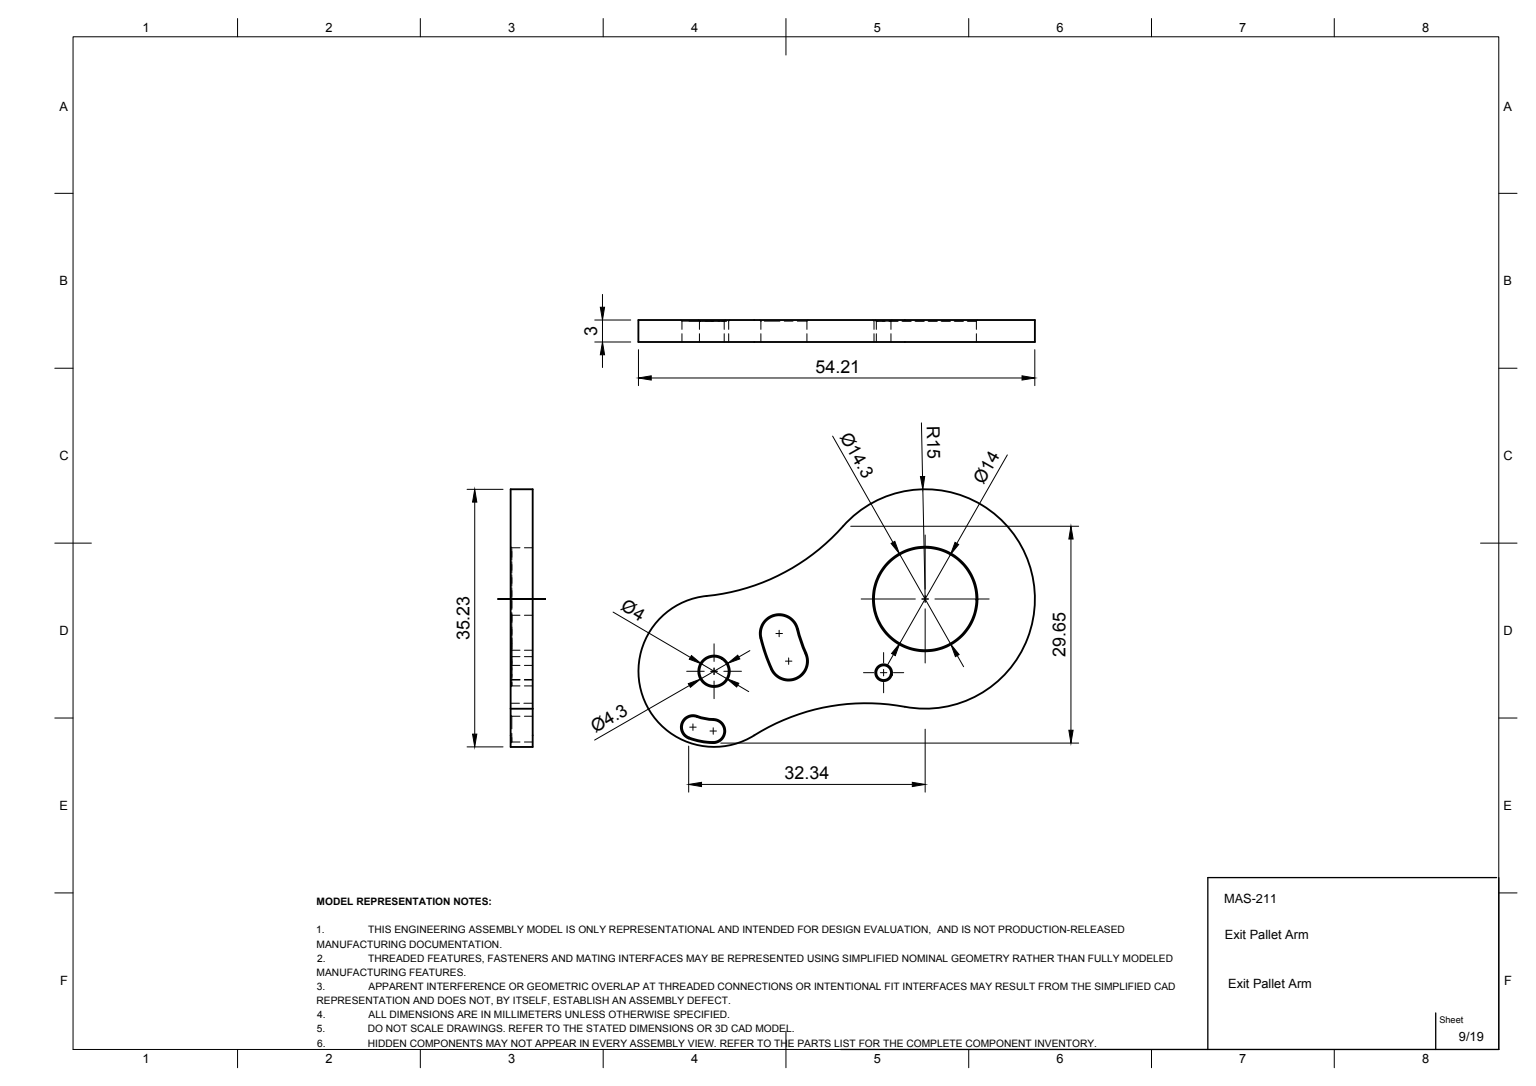
ISO-10303-21;
HEADER;
FILE_DESCRIPTION(
 (''),
 '2;1');
FILE_NAME ( 'Exit Pallet Arm.step', '2026-10-05T20:07:59+06:00', ( '' ), ( '' ), 'STEP AP214', 'Unspecified', '' );
FILE_SCHEMA (('AUTOMOTIVE_DESIGN { 1 0 10303 214 3 1 1 }'));
ENDSEC;
DATA;
#10=MECHANICAL_DESIGN_GEOMETRIC_PRESENTATION_REPRESENTATION('',(#326),#196741);
#135=ELLIPSE('',#8916,15.4840898354346,13.4083590350904) ;
#136=ELLIPSE('',#8917,20.0777465510709,17.3862071407216) ;
#137=ELLIPSE('',#8918,8.52758470717412,7.38293667736543) ;
#138=ELLIPSE('',#8919,5.66235729881268,4.90229438477269) ;
#326=STYLED_ITEM('',(#196765),#345) ;
#345=MANIFOLD_SOLID_BREP('Exit Pallet Arm',#8722) ;
#387=PLANE('',#8903) ;
#388=PLANE('',#8915) ;
#576=FACE_BOUND('',#1481,.T.) ;
#577=FACE_BOUND('',#1482,.T.) ;
#578=FACE_BOUND('',#1483,.T.) ;
#579=FACE_BOUND('',#1484,.T.) ;
#580=FACE_BOUND('',#1485,.T.) ;
#581=FACE_BOUND('',#1487,.T.) ;
#582=FACE_BOUND('',#1488,.T.) ;
#583=FACE_BOUND('',#1489,.T.) ;
#584=FACE_BOUND('',#1490,.T.) ;
#585=FACE_BOUND('',#1491,.T.) ;
#664=CIRCLE('',#8892,28.7407375552556) ;
#665=CIRCLE('',#8893,28.7407375552556) ;
#666=CIRCLE('',#8895,15.) ;
#667=CIRCLE('',#8896,15.) ;
#668=CIRCLE('',#8898,28.7407375552573) ;
#669=CIRCLE('',#8899,28.7407375552573) ;
#670=CIRCLE('',#8901,10.3432265401781) ;
#671=CIRCLE('',#8902,10.3432265401781) ;
#672=CIRCLE('',#8904,2.) ;
#673=CIRCLE('',#8905,23.0149881946393) ;
#674=CIRCLE('',#8906,2.4999999999999) ;
#675=CIRCLE('',#8907,18.0149881946822) ;
#676=CIRCLE('',#8908,2.49999999999984) ;
#677=CIRCLE('',#8909,7.) ;
#678=CIRCLE('',#8910,1.49999999999999) ;
#679=CIRCLE('',#8911,6.67161327010524) ;
#680=CIRCLE('',#8912,1.49999999999977) ;
#681=CIRCLE('',#8913,9.67161327008901) ;
#682=CIRCLE('',#8914,0.999999999999985) ;
#683=CIRCLE('',#8921,2.00000000000002) ;
#684=CIRCLE('',#8924,18.0149881946818) ;
#685=CIRCLE('',#8928,7.) ;
#686=CIRCLE('',#8932,6.67161327010476) ;
#846=B_SPLINE_SURFACE_WITH_KNOTS('',3,1,((#113566,#113567),(#113568,#113569),
(#113570,#113571),(#113572,#113573),(#113574,#113575),(#113576,#113577),
(#113578,#113579),(#113580,#113581),(#113582,#113583),(#113584,#113585),
(#113586,#113587),(#113588,#113589),(#113590,#113591),(#113592,#113593),
(#113594,#113595),(#113596,#113597),(#113598,#113599),(#113600,#113601),
(#113602,#113603)),.UNSPECIFIED.,.T.,.F.,.F.,(4,1,1,1,1,1,1,1,1,1,1,1,1,
1,1,1,4),(2,2),(0.,0.844281694673181,1.68856338934636,2.5328450840081,3.37712677866985,
4.22140847333585,5.06569016800186,5.90997186266359,6.75425355732532,7.59853525198361,
8.44281694664191,9.28709864130793,10.131380335974,10.9756620306357,11.8199437252974,
12.6642254199629,13.5085071146283),(-0.0112712723182462,0.214916064351496),
 .UNSPECIFIED.) ;
#847=B_SPLINE_SURFACE_WITH_KNOTS('',3,1,((#113605,#113606),(#113607,#113608),
(#113609,#113610),(#113611,#113612),(#113613,#113614),(#113615,#113616),
(#113617,#113618),(#113619,#113620),(#113621,#113622),(#113623,#113624),
(#113625,#113626)),.UNSPECIFIED.,.F.,.F.,.F.,(4,1,1,1,1,1,1,1,4),(2,2),
(0.,1.04064620349252,2.08129240698504,3.12193860704037,4.16258480709569,
5.20323100714621,6.24387720719672,7.28452341068925,8.32516961418178),(0.,
0.214915892305322),.UNSPECIFIED.) ;
#848=B_SPLINE_SURFACE_WITH_KNOTS('',3,1,((#113629,#113630),(#113631,#113632),
(#113633,#113634),(#113635,#113636)),.UNSPECIFIED.,.F.,.F.,.F.,(4,4),(2,
2),(-1.11022302462516E-16,3.4846841528001),(0.,0.212356567860235),
 .UNSPECIFIED.) ;
#849=B_SPLINE_SURFACE_WITH_KNOTS('',3,1,((#113638,#113639),(#113640,#113641),
(#113642,#113643),(#113644,#113645),(#113646,#113647),(#113648,#113649),
(#113650,#113651),(#113652,#113653),(#113654,#113655),(#113656,#113657),
(#113658,#113659)),.UNSPECIFIED.,.F.,.F.,.F.,(4,1,1,1,1,1,1,1,4),(2,2),
(0.,1.04062614942688,2.08125229885376,3.12187844827613,4.1625045976985,
5.20313074711665,6.24375689653479,7.28438304596787,8.32500919540094),(0.,
0.214916063344399),.UNSPECIFIED.) ;
#850=B_SPLINE_SURFACE_WITH_KNOTS('',3,1,((#113661,#113662),(#113663,#113664),
(#113665,#113666),(#113667,#113668)),.UNSPECIFIED.,.F.,.F.,.F.,(4,4),(2,
2),(-1.11022302462516E-16,4.5184839002944),(-6.99189761287855E-5,0.212356567829033),
 .UNSPECIFIED.) ;
#851=B_SPLINE_SURFACE_WITH_KNOTS('',3,1,((#113669,#113670),(#113671,#113672),
(#113673,#113674),(#113675,#113676),(#113677,#113678),(#113679,#113680),
(#113681,#113682),(#113683,#113684),(#113685,#113686),(#113687,#113688),
(#113689,#113690),(#113691,#113692),(#113693,#113694),(#113695,#113696),
(#113697,#113698),(#113699,#113700),(#113701,#113702),(#113703,#113704),
(#113705,#113706)),.UNSPECIFIED.,.T.,.F.,.F.,(4,1,1,1,1,1,1,1,1,1,1,1,1,
1,1,1,4),(2,2),(0.,2.69519445779222,5.61545499238395,8.53571552697321,11.2309099847624,
13.9261044425516,16.8463649771433,19.7666255117326,22.4618199695217,25.1570144273109,
28.0772749619002,30.9975354964919,33.692729954281,36.3879244120702,39.3081849466595,
42.2284454812513,44.9236399390404),(-0.0215150649611441,0.215150649611441),
 .UNSPECIFIED.) ;
#852=B_SPLINE_SURFACE_WITH_KNOTS('',3,1,((#113708,#113709),(#113710,#113711),
(#113712,#113713),(#113714,#113715)),.UNSPECIFIED.,.F.,.F.,.F.,(4,4),(2,
2),(-1.20032081259135E-14,3.40704145701401),(-0.000292137134752522,0.212844506430324),
 .UNSPECIFIED.) ;
#853=B_SPLINE_SURFACE_WITH_KNOTS('',3,1,((#113718,#113719),(#113720,#113721),
(#113722,#113723),(#113724,#113725),(#113726,#113727),(#113728,#113729),
(#113730,#113731),(#113732,#113733),(#113734,#113735)),.UNSPECIFIED.,.F.,
 .F.,.F.,(4,1,1,1,1,1,4),(2,2),(0.,1.2958739093245,1.94381087119137,2.59174783305825,
3.23968479492247,3.88762175678669,5.18349566611894),(0.,0.218727515290808),
 .UNSPECIFIED.) ;
#854=B_SPLINE_SURFACE_WITH_KNOTS('',3,1,((#113737,#113738),(#113739,#113740),
(#113741,#113742),(#113743,#113744)),.UNSPECIFIED.,.F.,.F.,.F.,(4,4),(2,
2),(0.,2.26229870547723),(0.,0.212844507129729),.UNSPECIFIED.) ;
#855=B_SPLINE_SURFACE_WITH_KNOTS('',3,1,((#113746,#113747),(#113748,#113749),
(#113750,#113751),(#113752,#113753),(#113754,#113755),(#113756,#113757),
(#113758,#113759),(#113760,#113761),(#113762,#113763)),.UNSPECIFIED.,.F.,
 .F.,.F.,(4,1,1,1,1,1,4),(2,2),(0.,1.29587422179652,1.94381133989956,2.5917484580026,
3.23968557610299,3.88762269420339,5.18349691602093),(0.,0.21872751905286),
 .UNSPECIFIED.) ;
#856=B_SPLINE_SURFACE_WITH_KNOTS('',3,1,((#113764,#113765),(#113766,#113767),
(#113768,#113769),(#113770,#113771),(#113772,#113773),(#113774,#113775),
(#113776,#113777),(#113778,#113779),(#113780,#113781),(#113782,#113783),
(#113784,#113785)),.UNSPECIFIED.,.T.,.F.,.F.,(4,1,1,1,1,1,1,1,4),(2,2),
(0.,0.903185063809554,1.80637013757091,2.70955520128371,3.61274027504511,
4.51592534880276,5.4191104125156,6.32229548627704,7.22548054998985),(0.,
0.223990409920864),.UNSPECIFIED.) ;
#981=FACE_OUTER_BOUND('',#1476,.T.) ;
#982=FACE_OUTER_BOUND('',#1477,.T.) ;
#983=FACE_OUTER_BOUND('',#1478,.T.) ;
#984=FACE_OUTER_BOUND('',#1479,.T.) ;
#985=FACE_OUTER_BOUND('',#1480,.T.) ;
#986=FACE_OUTER_BOUND('',#1486,.T.) ;
#987=FACE_OUTER_BOUND('',#1492,.T.) ;
#988=FACE_OUTER_BOUND('',#1493,.T.) ;
#989=FACE_OUTER_BOUND('',#1494,.T.) ;
#990=FACE_OUTER_BOUND('',#1495,.T.) ;
#991=FACE_OUTER_BOUND('',#1496,.T.) ;
#992=FACE_OUTER_BOUND('',#1497,.T.) ;
#993=FACE_OUTER_BOUND('',#1498,.T.) ;
#994=FACE_OUTER_BOUND('',#1499,.T.) ;
#995=FACE_OUTER_BOUND('',#1500,.T.) ;
#996=FACE_OUTER_BOUND('',#1501,.T.) ;
#997=FACE_OUTER_BOUND('',#1502,.T.) ;
#998=FACE_OUTER_BOUND('',#1503,.T.) ;
#999=FACE_OUTER_BOUND('',#1504,.T.) ;
#1000=FACE_OUTER_BOUND('',#1505,.T.) ;
#1001=FACE_OUTER_BOUND('',#1506,.T.) ;
#1002=FACE_OUTER_BOUND('',#1507,.T.) ;
#1003=FACE_OUTER_BOUND('',#1508,.T.) ;
#1004=FACE_OUTER_BOUND('',#1509,.T.) ;
#1005=FACE_OUTER_BOUND('',#1510,.T.) ;
#1006=FACE_OUTER_BOUND('',#1511,.T.) ;
#1007=FACE_OUTER_BOUND('',#1512,.T.) ;
#1008=FACE_OUTER_BOUND('',#1513,.T.) ;
#1476=EDGE_LOOP('',(#6216,#6217,#6218,#6219)) ;
#1477=EDGE_LOOP('',(#6220,#6221,#6222,#6223)) ;
#1478=EDGE_LOOP('',(#6224,#6225,#6226,#6227)) ;
#1479=EDGE_LOOP('',(#6228,#6229,#6230,#6231)) ;
#1480=EDGE_LOOP('',(#6232,#6233,#6234,#6235)) ;
#1481=EDGE_LOOP('',(#6236)) ;
#1482=EDGE_LOOP('',(#6237,#6238,#6239,#6240)) ;
#1483=EDGE_LOOP('',(#6241)) ;
#1484=EDGE_LOOP('',(#6242,#6243,#6244,#6245)) ;
#1485=EDGE_LOOP('',(#6246)) ;
#1486=EDGE_LOOP('',(#6247,#6248,#6249,#6250)) ;
#1487=EDGE_LOOP('',(#6251)) ;
#1488=EDGE_LOOP('',(#6252,#6253,#6254,#6255)) ;
#1489=EDGE_LOOP('',(#6256)) ;
#1490=EDGE_LOOP('',(#6257,#6258,#6259,#6260)) ;
#1491=EDGE_LOOP('',(#6261)) ;
#1492=EDGE_LOOP('',(#6262,#6263,#6264,#6265)) ;
#1493=EDGE_LOOP('',(#6266,#6267,#6268,#6269)) ;
#1494=EDGE_LOOP('',(#6270,#6271,#6272,#6273)) ;
#1495=EDGE_LOOP('',(#6274,#6275,#6276,#6277)) ;
#1496=EDGE_LOOP('',(#6278,#6279,#6280,#6281)) ;
#1497=EDGE_LOOP('',(#6282,#6283,#6284,#6285)) ;
#1498=EDGE_LOOP('',(#6286,#6287,#6288,#6289)) ;
#1499=EDGE_LOOP('',(#6290,#6291,#6292,#6293)) ;
#1500=EDGE_LOOP('',(#6294,#6295,#6296,#6297)) ;
#1501=EDGE_LOOP('',(#6298,#6299,#6300,#6301)) ;
#1502=EDGE_LOOP('',(#6302,#6303,#6304,#6305)) ;
#1503=EDGE_LOOP('',(#6306,#6307,#6308,#6309)) ;
#1504=EDGE_LOOP('',(#6310,#6311,#6312,#6313)) ;
#1505=EDGE_LOOP('',(#6314,#6315,#6316,#6317)) ;
#1506=EDGE_LOOP('',(#6318,#6319,#6320,#6321)) ;
#1507=EDGE_LOOP('',(#6322,#6323,#6324,#6325)) ;
#1508=EDGE_LOOP('',(#6326,#6327,#6328,#6329)) ;
#1509=EDGE_LOOP('',(#6330,#6331,#6332,#6333)) ;
#1510=EDGE_LOOP('',(#6334,#6335,#6336,#6337)) ;
#1511=EDGE_LOOP('',(#6338,#6339,#6340,#6341)) ;
#1512=EDGE_LOOP('',(#6342,#6343,#6344,#6345)) ;
#1513=EDGE_LOOP('',(#6346,#6347,#6348,#6349)) ;
#1981=LINE('',#113319,#2684) ;
#1982=LINE('',#113322,#2685) ;
#1983=LINE('',#113327,#2686) ;
#1984=LINE('',#113333,#2687) ;
#1985=LINE('',#113469,#2688) ;
#1986=LINE('',#113472,#2689) ;
#1987=LINE('',#113474,#2690) ;
#1988=LINE('',#113488,#2691) ;
#1989=LINE('',#113492,#2692) ;
#1990=LINE('',#113514,#2693) ;
#1991=LINE('',#113517,#2694) ;
#1992=LINE('',#113519,#2695) ;
#1993=LINE('',#113528,#2696) ;
#1994=LINE('',#113540,#2697) ;
#1995=LINE('',#113565,#2698) ;
#1996=LINE('',#113604,#2699) ;
#1997=LINE('',#113627,#2700) ;
#1998=LINE('',#113628,#2701) ;
#1999=LINE('',#113637,#2702) ;
#2000=LINE('',#113660,#2703) ;
#2001=LINE('',#113707,#2704) ;
#2002=LINE('',#113716,#2705) ;
#2003=LINE('',#113717,#2706) ;
#2004=LINE('',#113736,#2707) ;
#2005=LINE('',#113745,#2708) ;
#2006=LINE('',#113786,#2709) ;
#2684=VECTOR('',#9867,10.) ;
#2685=VECTOR('',#9870,10.) ;
#2686=VECTOR('',#9875,10.) ;
#2687=VECTOR('',#9882,10.) ;
#2688=VECTOR('',#9929,2.) ;
#2689=VECTOR('',#9932,10.) ;
#2690=VECTOR('',#9933,10.) ;
#2691=VECTOR('',#9936,10.) ;
#2692=VECTOR('',#9941,10.) ;
#2693=VECTOR('',#9948,6.99999999999998) ;
#2694=VECTOR('',#9951,10.) ;
#2695=VECTOR('',#9952,10.) ;
#2696=VECTOR('',#9955,10.) ;
#2697=VECTOR('',#9958,10.) ;
#2698=VECTOR('',#9965,0.999999999999981) ;
#2699=VECTOR('',#9966,10.) ;
#2700=VECTOR('',#9967,10.) ;
#2701=VECTOR('',#9968,10.) ;
#2702=VECTOR('',#9969,10.) ;
#2703=VECTOR('',#9970,10.) ;
#2704=VECTOR('',#9971,10.) ;
#2705=VECTOR('',#9972,10.) ;
#2706=VECTOR('',#9973,10.) ;
#2707=VECTOR('',#9974,10.) ;
#2708=VECTOR('',#9975,10.) ;
#2709=VECTOR('',#9976,10.) ;
#3419=B_SPLINE_CURVE_WITH_KNOTS('',3,(#113363,#113364,#113365,#113366,#113367,
#113368,#113369,#113370,#113371,#113372,#113373,#113374,#113375,#113376,
#113377,#113378,#113379,#113380,#113381),.UNSPECIFIED.,.T.,.F.,(4,1,1,1,
1,1,1,1,1,1,1,1,1,1,1,1,4),(0.,2.69519445779222,5.61545499238395,8.53571552697321,
11.2309099847624,13.9261044425516,16.8463649771433,19.7666255117326,22.4618199695217,
25.1570144273109,28.0772749619002,30.9975354964919,33.692729954281,36.3879244120702,
39.3081849466595,42.2284454812513,44.9236399390404),.UNSPECIFIED.) ;
#3420=B_SPLINE_CURVE_WITH_KNOTS('',3,(#113384,#113385,#113386,#113387,#113388,
#113389,#113390,#113391,#113392,#113393,#113394),.UNSPECIFIED.,.F.,.F.,
(4,1,1,1,1,1,1,1,4),(0.,1.04064620349252,2.08129240698504,3.12193860704037,
4.16258480709569,5.20323100714621,6.24387720719672,7.28452341068925,8.32516961418178),
 .UNSPECIFIED.) ;
#3421=B_SPLINE_CURVE_WITH_KNOTS('',3,(#113398,#113399,#113400,#113401,#113402,
#113403,#113404,#113405,#113406,#113407,#113408),.UNSPECIFIED.,.F.,.F.,
(4,1,1,1,1,1,1,1,4),(0.,1.04062614942688,2.08125229885376,3.12187844827613,
4.1625045976985,5.20313074711665,6.24375689653479,7.28438304596787,8.32500919540094),
 .UNSPECIFIED.) ;
#3422=B_SPLINE_CURVE_WITH_KNOTS('',3,(#113411,#113412,#113413,#113414,#113415,
#113416,#113417,#113418,#113419,#113420,#113421),.UNSPECIFIED.,.T.,.F.,
(4,1,1,1,1,1,1,1,4),(0.,0.903185063809554,1.80637013757091,2.70955520128371,
3.61274027504511,4.51592534880276,5.4191104125156,6.32229548627704,7.22548054998985),
 .UNSPECIFIED.) ;
#3423=B_SPLINE_CURVE_WITH_KNOTS('',3,(#113426,#113427,#113428,#113429,#113430,
#113431,#113432,#113433,#113434),.UNSPECIFIED.,.F.,.F.,(4,1,1,1,1,1,4),
(0.,1.2958739093245,1.94381087119137,2.59174783305825,3.23968479492247,
3.88762175678669,5.18349566611894),.UNSPECIFIED.) ;
#3424=B_SPLINE_CURVE_WITH_KNOTS('',3,(#113437,#113438,#113439,#113440,#113441,
#113442,#113443,#113444,#113445),.UNSPECIFIED.,.F.,.F.,(4,1,1,1,1,1,4),
(0.,1.29587422179652,1.94381133989956,2.5917484580026,3.23968557610299,
3.88762269420339,5.18349691602093),.UNSPECIFIED.) ;
#3425=B_SPLINE_CURVE_WITH_KNOTS('',3,(#113447,#113448,#113449,#113450,#113451,
#113452,#113453,#113454,#113455,#113456,#113457,#113458,#113459,#113460,
#113461,#113462,#113463,#113464,#113465),.UNSPECIFIED.,.T.,.F.,(4,1,1,1,
1,1,1,1,1,1,1,1,1,1,1,1,4),(0.,0.844281694673181,1.68856338934636,2.5328450840081,
3.37712677866985,4.22140847333585,5.06569016800186,5.90997186266359,6.75425355732532,
7.59853525198361,8.44281694664191,9.28709864130793,10.131380335974,10.9756620306357,
11.8199437252974,12.6642254199629,13.5085071146283),.UNSPECIFIED.) ;
#3426=B_SPLINE_CURVE_WITH_KNOTS('',3,(#113475,#113476,#113477,#113478,#113479,
#113480,#113481,#113482,#113483,#113484,#113485),.UNSPECIFIED.,.F.,.F.,
(4,1,1,1,1,1,1,1,4),(0.,1.04064620349252,2.08129240698504,3.12193860704037,
4.16258480709569,5.20323100714621,6.24387720719672,7.28452341068925,8.32516961418178),
 .UNSPECIFIED.) ;
#3427=B_SPLINE_CURVE_WITH_KNOTS('',3,(#113493,#113494,#113495,#113496,#113497,
#113498,#113499,#113500,#113501,#113502,#113503),.UNSPECIFIED.,.F.,.F.,
(4,1,1,1,1,1,1,1,4),(0.,1.04062614942688,2.08125229885376,3.12187844827613,
4.1625045976985,5.20313074711665,6.24375689653479,7.28438304596787,8.32500919540094),
 .UNSPECIFIED.) ;
#3428=B_SPLINE_CURVE_WITH_KNOTS('',3,(#113505,#113506,#113507,#113508,#113509,
#113510),.UNSPECIFIED.,.F.,.F.,(4,2,4),(0.,0.224505556318748,0.449011112637672),
 .UNSPECIFIED.) ;
#3429=B_SPLINE_CURVE_WITH_KNOTS('',3,(#113520,#113521,#113522,#113523,#113524,
#113525),.UNSPECIFIED.,.F.,.F.,(4,2,4),(0.,0.167853741155252,0.335707418129887),
 .UNSPECIFIED.) ;
#3430=B_SPLINE_CURVE_WITH_KNOTS('',3,(#113529,#113530,#113531,#113532,#113533,
#113534,#113535,#113536,#113537),.UNSPECIFIED.,.F.,.F.,(4,1,1,1,1,1,4),
(1.46151310183612E-7,1.2958739093245,1.94381087119137,2.59174783305825,
3.23968479492247,3.88762175678669,5.18349566611894),.UNSPECIFIED.) ;
#3431=B_SPLINE_CURVE_WITH_KNOTS('',3,(#113543,#113544,#113545,#113546,#113547,
#113548,#113549,#113550,#113551),.UNSPECIFIED.,.F.,.F.,(4,1,1,1,1,1,4),
(0.,1.29587422179652,1.94381133989956,2.5917484580026,3.23968557610299,
3.88762269420339,5.18349691602093),.UNSPECIFIED.) ;
#3432=B_SPLINE_CURVE_WITH_KNOTS('',3,(#113554,#113555,#113556,#113557,#113558,
#113559,#113560,#113561,#113562,#113563,#113564),.UNSPECIFIED.,.T.,.F.,
(4,1,1,1,1,1,1,1,4),(0.,0.903185063809554,1.80637013757091,2.70955520128371,
3.61274027504511,4.51592534880276,5.4191104125156,6.32229548627704,7.22548054998985),
 .UNSPECIFIED.) ;
#3663=VERTEX_POINT('',#113315) ;
#3664=VERTEX_POINT('',#113316) ;
#3665=VERTEX_POINT('',#113318) ;
#3666=VERTEX_POINT('',#113320) ;
#3667=VERTEX_POINT('',#113324) ;
#3668=VERTEX_POINT('',#113326) ;
#3669=VERTEX_POINT('',#113330) ;
#3670=VERTEX_POINT('',#113332) ;
#3671=VERTEX_POINT('',#113339) ;
#3672=VERTEX_POINT('',#113341) ;
#3673=VERTEX_POINT('',#113342) ;
#3674=VERTEX_POINT('',#113344) ;
#3675=VERTEX_POINT('',#113346) ;
#3676=VERTEX_POINT('',#113349) ;
#3677=VERTEX_POINT('',#113351) ;
#3678=VERTEX_POINT('',#113352) ;
#3679=VERTEX_POINT('',#113354) ;
#3680=VERTEX_POINT('',#113356) ;
#3681=VERTEX_POINT('',#113359) ;
#3682=VERTEX_POINT('',#113362) ;
#3683=VERTEX_POINT('',#113382) ;
#3684=VERTEX_POINT('',#113383) ;
#3685=VERTEX_POINT('',#113395) ;
#3686=VERTEX_POINT('',#113397) ;
#3687=VERTEX_POINT('',#113410) ;
#3688=VERTEX_POINT('',#113422) ;
#3689=VERTEX_POINT('',#113423) ;
#3690=VERTEX_POINT('',#113425) ;
#3691=VERTEX_POINT('',#113435) ;
#3692=VERTEX_POINT('',#113446) ;
#3693=VERTEX_POINT('',#113467) ;
#3694=VERTEX_POINT('',#113471) ;
#3695=VERTEX_POINT('',#113473) ;
#3696=VERTEX_POINT('',#113487) ;
#3697=VERTEX_POINT('',#113491) ;
#3698=VERTEX_POINT('',#113512) ;
#3699=VERTEX_POINT('',#113516) ;
#3700=VERTEX_POINT('',#113518) ;
#3701=VERTEX_POINT('',#113527) ;
#3702=VERTEX_POINT('',#113539) ;
#3703=VERTEX_POINT('',#113553) ;
#4616=EDGE_CURVE('',#3663,#3664,#664,.T.) ;
#4617=EDGE_CURVE('',#3664,#3665,#1981,.T.) ;
#4618=EDGE_CURVE('',#3666,#3665,#665,.T.) ;
#4619=EDGE_CURVE('',#3663,#3666,#1982,.T.) ;
#4620=EDGE_CURVE('',#3664,#3667,#666,.T.) ;
#4621=EDGE_CURVE('',#3667,#3668,#1983,.T.) ;
#4622=EDGE_CURVE('',#3665,#3668,#667,.T.) ;
#4623=EDGE_CURVE('',#3667,#3669,#668,.T.) ;
#4624=EDGE_CURVE('',#3669,#3670,#1984,.T.) ;
#4625=EDGE_CURVE('',#3668,#3670,#669,.T.) ;
#4626=EDGE_CURVE('',#3669,#3663,#670,.T.) ;
#4627=EDGE_CURVE('',#3670,#3666,#671,.T.) ;
#4628=EDGE_CURVE('',#3671,#3671,#672,.T.) ;
#4629=EDGE_CURVE('',#3672,#3673,#673,.T.) ;
#4630=EDGE_CURVE('',#3674,#3672,#674,.T.) ;
#4631=EDGE_CURVE('',#3675,#3674,#675,.T.) ;
#4632=EDGE_CURVE('',#3673,#3675,#676,.T.) ;
#4633=EDGE_CURVE('',#3676,#3676,#677,.T.) ;
#4634=EDGE_CURVE('',#3677,#3678,#678,.T.) ;
#4635=EDGE_CURVE('',#3679,#3677,#679,.T.) ;
#4636=EDGE_CURVE('',#3680,#3679,#680,.T.) ;
#4637=EDGE_CURVE('',#3678,#3680,#681,.T.) ;
#4638=EDGE_CURVE('',#3681,#3681,#682,.T.) ;
#4639=EDGE_CURVE('',#3682,#3682,#3419,.T.) ;
#4640=EDGE_CURVE('',#3683,#3684,#3420,.T.) ;
#4641=EDGE_CURVE('',#3684,#3685,#135,.T.) ;
#4642=EDGE_CURVE('',#3685,#3686,#3421,.T.) ;
#4643=EDGE_CURVE('',#3686,#3683,#136,.T.) ;
#4644=EDGE_CURVE('',#3687,#3687,#3422,.T.) ;
#4645=EDGE_CURVE('',#3688,#3689,#137,.T.) ;
#4646=EDGE_CURVE('',#3689,#3690,#3423,.T.) ;
#4647=EDGE_CURVE('',#3690,#3691,#138,.T.) ;
#4648=EDGE_CURVE('',#3691,#3688,#3424,.T.) ;
#4649=EDGE_CURVE('',#3692,#3692,#3425,.T.) ;
#4650=EDGE_CURVE('',#3693,#3693,#683,.T.) ;
#4651=EDGE_CURVE('',#3693,#3671,#1985,.T.) ;
#4652=EDGE_CURVE('',#3673,#3694,#1986,.T.) ;
#4653=EDGE_CURVE('',#3675,#3695,#1987,.T.) ;
#4654=EDGE_CURVE('',#3694,#3695,#3426,.T.) ;
#4655=EDGE_CURVE('',#3674,#3696,#1988,.T.) ;
#4656=EDGE_CURVE('',#3695,#3696,#684,.T.) ;
#4657=EDGE_CURVE('',#3672,#3697,#1989,.T.) ;
#4658=EDGE_CURVE('',#3696,#3697,#3427,.T.) ;
#4659=EDGE_CURVE('',#3697,#3694,#3428,.T.) ;
#4660=EDGE_CURVE('',#3698,#3698,#685,.T.) ;
#4661=EDGE_CURVE('',#3698,#3676,#1990,.T.) ;
#4662=EDGE_CURVE('',#3678,#3699,#1991,.T.) ;
#4663=EDGE_CURVE('',#3680,#3700,#1992,.T.) ;
#4664=EDGE_CURVE('',#3699,#3700,#3429,.T.) ;
#4665=EDGE_CURVE('',#3679,#3701,#1993,.T.) ;
#4666=EDGE_CURVE('',#3700,#3701,#3430,.T.) ;
#4667=EDGE_CURVE('',#3677,#3702,#1994,.T.) ;
#4668=EDGE_CURVE('',#3701,#3702,#686,.T.) ;
#4669=EDGE_CURVE('',#3702,#3699,#3431,.T.) ;
#4670=EDGE_CURVE('',#3703,#3703,#3432,.T.) ;
#4671=EDGE_CURVE('',#3703,#3681,#1995,.T.) ;
#4672=EDGE_CURVE('',#3693,#3692,#1996,.T.) ;
#4673=EDGE_CURVE('',#3695,#3684,#1997,.T.) ;
#4674=EDGE_CURVE('',#3683,#3694,#1998,.T.) ;
#4675=EDGE_CURVE('',#3696,#3685,#1999,.T.) ;
#4676=EDGE_CURVE('',#3697,#3686,#2000,.T.) ;
#4677=EDGE_CURVE('',#3698,#3682,#2001,.T.) ;
#4678=EDGE_CURVE('',#3700,#3689,#2002,.T.) ;
#4679=EDGE_CURVE('',#3699,#3688,#2003,.T.) ;
#4680=EDGE_CURVE('',#3701,#3690,#2004,.T.) ;
#4681=EDGE_CURVE('',#3702,#3691,#2005,.T.) ;
#4682=EDGE_CURVE('',#3703,#3687,#2006,.T.) ;
#6216=ORIENTED_EDGE('',*,*,#4616,.T.) ;
#6217=ORIENTED_EDGE('',*,*,#4617,.T.) ;
#6218=ORIENTED_EDGE('',*,*,#4618,.F.) ;
#6219=ORIENTED_EDGE('',*,*,#4619,.F.) ;
#6220=ORIENTED_EDGE('',*,*,#4620,.T.) ;
#6221=ORIENTED_EDGE('',*,*,#4621,.T.) ;
#6222=ORIENTED_EDGE('',*,*,#4622,.F.) ;
#6223=ORIENTED_EDGE('',*,*,#4617,.F.) ;
#6224=ORIENTED_EDGE('',*,*,#4623,.T.) ;
#6225=ORIENTED_EDGE('',*,*,#4624,.T.) ;
#6226=ORIENTED_EDGE('',*,*,#4625,.F.) ;
#6227=ORIENTED_EDGE('',*,*,#4621,.F.) ;
#6228=ORIENTED_EDGE('',*,*,#4626,.T.) ;
#6229=ORIENTED_EDGE('',*,*,#4619,.T.) ;
#6230=ORIENTED_EDGE('',*,*,#4627,.F.) ;
#6231=ORIENTED_EDGE('',*,*,#4624,.F.) ;
#6232=ORIENTED_EDGE('',*,*,#4626,.F.) ;
#6233=ORIENTED_EDGE('',*,*,#4623,.F.) ;
#6234=ORIENTED_EDGE('',*,*,#4620,.F.) ;
#6235=ORIENTED_EDGE('',*,*,#4616,.F.) ;
#6236=ORIENTED_EDGE('',*,*,#4628,.F.) ;
#6237=ORIENTED_EDGE('',*,*,#4629,.F.) ;
#6238=ORIENTED_EDGE('',*,*,#4630,.F.) ;
#6239=ORIENTED_EDGE('',*,*,#4631,.F.) ;
#6240=ORIENTED_EDGE('',*,*,#4632,.F.) ;
#6241=ORIENTED_EDGE('',*,*,#4633,.F.) ;
#6242=ORIENTED_EDGE('',*,*,#4634,.F.) ;
#6243=ORIENTED_EDGE('',*,*,#4635,.F.) ;
#6244=ORIENTED_EDGE('',*,*,#4636,.F.) ;
#6245=ORIENTED_EDGE('',*,*,#4637,.F.) ;
#6246=ORIENTED_EDGE('',*,*,#4638,.F.) ;
#6247=ORIENTED_EDGE('',*,*,#4618,.T.) ;
#6248=ORIENTED_EDGE('',*,*,#4622,.T.) ;
#6249=ORIENTED_EDGE('',*,*,#4625,.T.) ;
#6250=ORIENTED_EDGE('',*,*,#4627,.T.) ;
#6251=ORIENTED_EDGE('',*,*,#4639,.T.) ;
#6252=ORIENTED_EDGE('',*,*,#4640,.T.) ;
#6253=ORIENTED_EDGE('',*,*,#4641,.T.) ;
#6254=ORIENTED_EDGE('',*,*,#4642,.T.) ;
#6255=ORIENTED_EDGE('',*,*,#4643,.T.) ;
#6256=ORIENTED_EDGE('',*,*,#4644,.T.) ;
#6257=ORIENTED_EDGE('',*,*,#4645,.T.) ;
#6258=ORIENTED_EDGE('',*,*,#4646,.T.) ;
#6259=ORIENTED_EDGE('',*,*,#4647,.T.) ;
#6260=ORIENTED_EDGE('',*,*,#4648,.T.) ;
#6261=ORIENTED_EDGE('',*,*,#4649,.T.) ;
#6262=ORIENTED_EDGE('',*,*,#4650,.F.) ;
#6263=ORIENTED_EDGE('',*,*,#4651,.T.) ;
#6264=ORIENTED_EDGE('',*,*,#4628,.T.) ;
#6265=ORIENTED_EDGE('',*,*,#4651,.F.) ;
#6266=ORIENTED_EDGE('',*,*,#4652,.F.) ;
#6267=ORIENTED_EDGE('',*,*,#4632,.T.) ;
#6268=ORIENTED_EDGE('',*,*,#4653,.T.) ;
#6269=ORIENTED_EDGE('',*,*,#4654,.F.) ;
#6270=ORIENTED_EDGE('',*,*,#4653,.F.) ;
#6271=ORIENTED_EDGE('',*,*,#4631,.T.) ;
#6272=ORIENTED_EDGE('',*,*,#4655,.T.) ;
#6273=ORIENTED_EDGE('',*,*,#4656,.F.) ;
#6274=ORIENTED_EDGE('',*,*,#4655,.F.) ;
#6275=ORIENTED_EDGE('',*,*,#4630,.T.) ;
#6276=ORIENTED_EDGE('',*,*,#4657,.T.) ;
#6277=ORIENTED_EDGE('',*,*,#4658,.F.) ;
#6278=ORIENTED_EDGE('',*,*,#4657,.F.) ;
#6279=ORIENTED_EDGE('',*,*,#4629,.T.) ;
#6280=ORIENTED_EDGE('',*,*,#4652,.T.) ;
#6281=ORIENTED_EDGE('',*,*,#4659,.F.) ;
#6282=ORIENTED_EDGE('',*,*,#4660,.F.) ;
#6283=ORIENTED_EDGE('',*,*,#4661,.T.) ;
#6284=ORIENTED_EDGE('',*,*,#4633,.T.) ;
#6285=ORIENTED_EDGE('',*,*,#4661,.F.) ;
#6286=ORIENTED_EDGE('',*,*,#4662,.F.) ;
#6287=ORIENTED_EDGE('',*,*,#4637,.T.) ;
#6288=ORIENTED_EDGE('',*,*,#4663,.T.) ;
#6289=ORIENTED_EDGE('',*,*,#4664,.F.) ;
#6290=ORIENTED_EDGE('',*,*,#4663,.F.) ;
#6291=ORIENTED_EDGE('',*,*,#4636,.T.) ;
#6292=ORIENTED_EDGE('',*,*,#4665,.T.) ;
#6293=ORIENTED_EDGE('',*,*,#4666,.F.) ;
#6294=ORIENTED_EDGE('',*,*,#4665,.F.) ;
#6295=ORIENTED_EDGE('',*,*,#4635,.T.) ;
#6296=ORIENTED_EDGE('',*,*,#4667,.T.) ;
#6297=ORIENTED_EDGE('',*,*,#4668,.F.) ;
#6298=ORIENTED_EDGE('',*,*,#4667,.F.) ;
#6299=ORIENTED_EDGE('',*,*,#4634,.T.) ;
#6300=ORIENTED_EDGE('',*,*,#4662,.T.) ;
#6301=ORIENTED_EDGE('',*,*,#4669,.F.) ;
#6302=ORIENTED_EDGE('',*,*,#4670,.F.) ;
#6303=ORIENTED_EDGE('',*,*,#4671,.T.) ;
#6304=ORIENTED_EDGE('',*,*,#4638,.T.) ;
#6305=ORIENTED_EDGE('',*,*,#4671,.F.) ;
#6306=ORIENTED_EDGE('',*,*,#4650,.T.) ;
#6307=ORIENTED_EDGE('',*,*,#4672,.T.) ;
#6308=ORIENTED_EDGE('',*,*,#4649,.F.) ;
#6309=ORIENTED_EDGE('',*,*,#4672,.F.) ;
#6310=ORIENTED_EDGE('',*,*,#4654,.T.) ;
#6311=ORIENTED_EDGE('',*,*,#4673,.T.) ;
#6312=ORIENTED_EDGE('',*,*,#4640,.F.) ;
#6313=ORIENTED_EDGE('',*,*,#4674,.T.) ;
#6314=ORIENTED_EDGE('',*,*,#4656,.T.) ;
#6315=ORIENTED_EDGE('',*,*,#4675,.T.) ;
#6316=ORIENTED_EDGE('',*,*,#4641,.F.) ;
#6317=ORIENTED_EDGE('',*,*,#4673,.F.) ;
#6318=ORIENTED_EDGE('',*,*,#4658,.T.) ;
#6319=ORIENTED_EDGE('',*,*,#4676,.T.) ;
#6320=ORIENTED_EDGE('',*,*,#4642,.F.) ;
#6321=ORIENTED_EDGE('',*,*,#4675,.F.) ;
#6322=ORIENTED_EDGE('',*,*,#4659,.T.) ;
#6323=ORIENTED_EDGE('',*,*,#4674,.F.) ;
#6324=ORIENTED_EDGE('',*,*,#4643,.F.) ;
#6325=ORIENTED_EDGE('',*,*,#4676,.F.) ;
#6326=ORIENTED_EDGE('',*,*,#4660,.T.) ;
#6327=ORIENTED_EDGE('',*,*,#4677,.T.) ;
#6328=ORIENTED_EDGE('',*,*,#4639,.F.) ;
#6329=ORIENTED_EDGE('',*,*,#4677,.F.) ;
#6330=ORIENTED_EDGE('',*,*,#4664,.T.) ;
#6331=ORIENTED_EDGE('',*,*,#4678,.T.) ;
#6332=ORIENTED_EDGE('',*,*,#4645,.F.) ;
#6333=ORIENTED_EDGE('',*,*,#4679,.F.) ;
#6334=ORIENTED_EDGE('',*,*,#4666,.T.) ;
#6335=ORIENTED_EDGE('',*,*,#4680,.T.) ;
#6336=ORIENTED_EDGE('',*,*,#4646,.F.) ;
#6337=ORIENTED_EDGE('',*,*,#4678,.F.) ;
#6338=ORIENTED_EDGE('',*,*,#4668,.T.) ;
#6339=ORIENTED_EDGE('',*,*,#4681,.T.) ;
#6340=ORIENTED_EDGE('',*,*,#4647,.F.) ;
#6341=ORIENTED_EDGE('',*,*,#4680,.F.) ;
#6342=ORIENTED_EDGE('',*,*,#4669,.T.) ;
#6343=ORIENTED_EDGE('',*,*,#4679,.T.) ;
#6344=ORIENTED_EDGE('',*,*,#4648,.F.) ;
#6345=ORIENTED_EDGE('',*,*,#4681,.F.) ;
#6346=ORIENTED_EDGE('',*,*,#4670,.T.) ;
#6347=ORIENTED_EDGE('',*,*,#4682,.T.) ;
#6348=ORIENTED_EDGE('',*,*,#4644,.F.) ;
#6349=ORIENTED_EDGE('',*,*,#4682,.F.) ;
#8169=CYLINDRICAL_SURFACE('',#8891,28.7407375552557) ;
#8170=CYLINDRICAL_SURFACE('',#8894,14.9999999999999) ;
#8171=CYLINDRICAL_SURFACE('',#8897,28.7407375552568) ;
#8172=CYLINDRICAL_SURFACE('',#8900,10.3432265401782) ;
#8173=CYLINDRICAL_SURFACE('',#8920,2.) ;
#8174=CYLINDRICAL_SURFACE('',#8922,2.49999999999952) ;
#8175=CYLINDRICAL_SURFACE('',#8923,18.014988194682) ;
#8176=CYLINDRICAL_SURFACE('',#8925,2.49999999999988) ;
#8177=CYLINDRICAL_SURFACE('',#8926,23.0149881946396) ;
#8178=CYLINDRICAL_SURFACE('',#8927,6.99999999999998) ;
#8179=CYLINDRICAL_SURFACE('',#8929,9.67161327008889) ;
#8180=CYLINDRICAL_SURFACE('',#8930,1.49999999999977) ;
#8181=CYLINDRICAL_SURFACE('',#8931,6.6716132701054) ;
#8182=CYLINDRICAL_SURFACE('',#8933,1.50000000000005) ;
#8183=CYLINDRICAL_SURFACE('',#8934,0.999999999999981) ;
#8364=ADVANCED_FACE('',(#981),#8169,.F.) ;
#8365=ADVANCED_FACE('',(#982),#8170,.T.) ;
#8366=ADVANCED_FACE('',(#983),#8171,.F.) ;
#8367=ADVANCED_FACE('',(#984),#8172,.T.) ;
#8368=ADVANCED_FACE('',(#985,#576,#577,#578,#579,#580),#387,.T.) ;
#8369=ADVANCED_FACE('',(#986,#581,#582,#583,#584,#585),#388,.T.) ;
#8370=ADVANCED_FACE('',(#987),#8173,.F.) ;
#8371=ADVANCED_FACE('',(#988),#8174,.F.) ;
#8372=ADVANCED_FACE('',(#989),#8175,.T.) ;
#8373=ADVANCED_FACE('',(#990),#8176,.F.) ;
#8374=ADVANCED_FACE('',(#991),#8177,.F.) ;
#8375=ADVANCED_FACE('',(#992),#8178,.F.) ;
#8376=ADVANCED_FACE('',(#993),#8179,.F.) ;
#8377=ADVANCED_FACE('',(#994),#8180,.F.) ;
#8378=ADVANCED_FACE('',(#995),#8181,.T.) ;
#8379=ADVANCED_FACE('',(#996),#8182,.F.) ;
#8380=ADVANCED_FACE('',(#997),#8183,.F.) ;
#8381=ADVANCED_FACE('',(#998),#846,.T.) ;
#8382=ADVANCED_FACE('',(#999),#847,.T.) ;
#8383=ADVANCED_FACE('',(#1000),#848,.T.) ;
#8384=ADVANCED_FACE('',(#1001),#849,.T.) ;
#8385=ADVANCED_FACE('',(#1002),#850,.T.) ;
#8386=ADVANCED_FACE('',(#1003),#851,.T.) ;
#8387=ADVANCED_FACE('',(#1004),#852,.T.) ;
#8388=ADVANCED_FACE('',(#1005),#853,.T.) ;
#8389=ADVANCED_FACE('',(#1006),#854,.T.) ;
#8390=ADVANCED_FACE('',(#1007),#855,.T.) ;
#8391=ADVANCED_FACE('',(#1008),#856,.T.) ;
#8722=CLOSED_SHELL('',(#8364,#8365,#8366,#8367,#8368,#8369,#8370,#8371,
#8372,#8373,#8374,#8375,#8376,#8377,#8378,#8379,#8380,#8381,#8382,#8383,
#8384,#8385,#8386,#8387,#8388,#8389,#8390,#8391)) ;
#8891=AXIS2_PLACEMENT_3D('',#113314,#9863,#9864) ;
#8892=AXIS2_PLACEMENT_3D('',#113317,#9865,#9866) ;
#8893=AXIS2_PLACEMENT_3D('',#113321,#9868,#9869) ;
#8894=AXIS2_PLACEMENT_3D('',#113323,#9871,#9872) ;
#8895=AXIS2_PLACEMENT_3D('',#113325,#9873,#9874) ;
#8896=AXIS2_PLACEMENT_3D('',#113328,#9876,#9877) ;
#8897=AXIS2_PLACEMENT_3D('',#113329,#9878,#9879) ;
#8898=AXIS2_PLACEMENT_3D('',#113331,#9880,#9881) ;
#8899=AXIS2_PLACEMENT_3D('',#113334,#9883,#9884) ;
#8900=AXIS2_PLACEMENT_3D('',#113335,#9885,#9886) ;
#8901=AXIS2_PLACEMENT_3D('',#113336,#9887,#9888) ;
#8902=AXIS2_PLACEMENT_3D('',#113337,#9889,#9890) ;
#8903=AXIS2_PLACEMENT_3D('',#113338,#9891,#9892) ;
#8904=AXIS2_PLACEMENT_3D('',#113340,#9893,#9894) ;
#8905=AXIS2_PLACEMENT_3D('',#113343,#9895,#9896) ;
#8906=AXIS2_PLACEMENT_3D('',#113345,#9897,#9898) ;
#8907=AXIS2_PLACEMENT_3D('',#113347,#9899,#9900) ;
#8908=AXIS2_PLACEMENT_3D('',#113348,#9901,#9902) ;
#8909=AXIS2_PLACEMENT_3D('',#113350,#9903,#9904) ;
#8910=AXIS2_PLACEMENT_3D('',#113353,#9905,#9906) ;
#8911=AXIS2_PLACEMENT_3D('',#113355,#9907,#9908) ;
#8912=AXIS2_PLACEMENT_3D('',#113357,#9909,#9910) ;
#8913=AXIS2_PLACEMENT_3D('',#113358,#9911,#9912) ;
#8914=AXIS2_PLACEMENT_3D('',#113360,#9913,#9914) ;
#8915=AXIS2_PLACEMENT_3D('',#113361,#9915,#9916) ;
#8916=AXIS2_PLACEMENT_3D('',#113396,#9917,#9918) ;
#8917=AXIS2_PLACEMENT_3D('',#113409,#9919,#9920) ;
#8918=AXIS2_PLACEMENT_3D('',#113424,#9921,#9922) ;
#8919=AXIS2_PLACEMENT_3D('',#113436,#9923,#9924) ;
#8920=AXIS2_PLACEMENT_3D('',#113466,#9925,#9926) ;
#8921=AXIS2_PLACEMENT_3D('',#113468,#9927,#9928) ;
#8922=AXIS2_PLACEMENT_3D('',#113470,#9930,#9931) ;
#8923=AXIS2_PLACEMENT_3D('',#113486,#9934,#9935) ;
#8924=AXIS2_PLACEMENT_3D('',#113489,#9937,#9938) ;
#8925=AXIS2_PLACEMENT_3D('',#113490,#9939,#9940) ;
#8926=AXIS2_PLACEMENT_3D('',#113504,#9942,#9943) ;
#8927=AXIS2_PLACEMENT_3D('',#113511,#9944,#9945) ;
#8928=AXIS2_PLACEMENT_3D('',#113513,#9946,#9947) ;
#8929=AXIS2_PLACEMENT_3D('',#113515,#9949,#9950) ;
#8930=AXIS2_PLACEMENT_3D('',#113526,#9953,#9954) ;
#8931=AXIS2_PLACEMENT_3D('',#113538,#9956,#9957) ;
#8932=AXIS2_PLACEMENT_3D('',#113541,#9959,#9960) ;
#8933=AXIS2_PLACEMENT_3D('',#113542,#9961,#9962) ;
#8934=AXIS2_PLACEMENT_3D('',#113552,#9963,#9964) ;
#9863=DIRECTION('center_axis',(0.,-1.,0.)) ;
#9864=DIRECTION('ref_axis',(-0.186143933560965,0.,0.982522486255888)) ;
#9865=DIRECTION('center_axis',(0.,1.,0.)) ;
#9866=DIRECTION('ref_axis',(0.184992222813461,0.,0.982739984684929)) ;
#9867=DIRECTION('',(0.,-1.,0.)) ;
#9868=DIRECTION('center_axis',(1.04405775373719E-16,1.,-5.51084421808798E-16)) ;
#9869=DIRECTION('ref_axis',(0.184992222813461,5.40804574512736E-16,0.982739984684929)) ;
#9870=DIRECTION('',(0.,-1.,0.)) ;
#9871=DIRECTION('center_axis',(0.,1.,0.)) ;
#9872=DIRECTION('ref_axis',(0.946102418141937,0.,0.323867587736069)) ;
#9873=DIRECTION('center_axis',(0.,-1.,0.)) ;
#9874=DIRECTION('ref_axis',(-0.748430942382017,0.,0.66321272943541)) ;
#9875=DIRECTION('',(0.,-1.,0.)) ;
#9876=DIRECTION('center_axis',(0.,-1.,0.)) ;
#9877=DIRECTION('ref_axis',(-0.748430942382017,0.,0.66321272943541)) ;
#9878=DIRECTION('center_axis',(0.,-1.,0.)) ;
#9879=DIRECTION('ref_axis',(0.455018599800648,0.,-0.890481933469432)) ;
#9880=DIRECTION('center_axis',(2.55214171167679E-16,1.,-4.99460041171418E-16)) ;
#9881=DIRECTION('ref_axis',(0.0989310425378922,-5.40804574512704E-16,-0.995094291422861)) ;
#9882=DIRECTION('',(0.,-1.,0.)) ;
#9883=DIRECTION('center_axis',(2.55214171167679E-16,1.,-4.99460041171418E-16)) ;
#9884=DIRECTION('ref_axis',(0.0989310425378922,-5.40804574512704E-16,-0.995094291422861)) ;
#9885=DIRECTION('center_axis',(0.,1.,0.)) ;
#9886=DIRECTION('ref_axis',(-0.946102418141937,0.,-0.323867587736068)) ;
#9887=DIRECTION('center_axis',(0.,-1.,0.)) ;
#9888=DIRECTION('ref_axis',(0.53164023528083,0.,-0.846970282967793)) ;
#9889=DIRECTION('center_axis',(0.,-1.,0.)) ;
#9890=DIRECTION('ref_axis',(0.53164023528083,0.,-0.846970282967793)) ;
#9891=DIRECTION('center_axis',(0.,1.,0.)) ;
#9892=DIRECTION('ref_axis',(0.,0.,1.)) ;
#9893=DIRECTION('center_axis',(0.,1.,0.)) ;
#9894=DIRECTION('ref_axis',(-0.0741867580339807,0.,0.997244365706023)) ;
#9895=DIRECTION('center_axis',(-9.60395745588678E-15,1.,-3.2876049804992E-15)) ;
#9896=DIRECTION('ref_axis',(-0.973142633081286,-1.00819783257896E-14,-0.230202987990212)) ;
#9897=DIRECTION('center_axis',(0.,1.,0.)) ;
#9898=DIRECTION('ref_axis',(-0.910070048017682,0.,-0.414454469997724)) ;
#9899=DIRECTION('center_axis',(0.,-1.,0.)) ;
#9900=DIRECTION('ref_axis',(-0.910070204982189,0.,-0.414454125330749)) ;
#9901=DIRECTION('center_axis',(0.,1.,0.)) ;
#9902=DIRECTION('ref_axis',(0.973142645774834,0.,0.230202934330464)) ;
#9903=DIRECTION('center_axis',(-7.09105905758385E-17,1.,5.21847544066181E-16)) ;
#9904=DIRECTION('ref_axis',(0.821909814783993,-3.1720657846433E-16,0.569617640493816)) ;
#9905=DIRECTION('center_axis',(-1.48015126885593E-15,1.,2.07969639555734E-17)) ;
#9906=DIRECTION('ref_axis',(-0.0140491798391936,0.,-0.999901305402611)) ;
#9907=DIRECTION('center_axis',(0.,-1.,0.)) ;
#9908=DIRECTION('ref_axis',(-0.0140491798343224,0.,-0.99990130540268)) ;
#9909=DIRECTION('center_axis',(1.38491428068804E-15,1.,-5.22775657039832E-16)) ;
#9910=DIRECTION('ref_axis',(0.353155349954092,0.,0.935564695143421)) ;
#9911=DIRECTION('center_axis',(1.42608153219998E-15,1.,7.51659194327274E-15)) ;
#9912=DIRECTION('ref_axis',(-0.353156058759361,7.57626650063376E-15,-0.935564427584522)) ;
#9913=DIRECTION('center_axis',(5.68566921680937E-16,1.,1.17837026301599E-17)) ;
#9914=DIRECTION('ref_axis',(0.945793391259251,0.,0.324768934860349)) ;
#9915=DIRECTION('center_axis',(0.,-1.,0.)) ;
#9916=DIRECTION('ref_axis',(0.,0.,-1.)) ;
#9917=DIRECTION('center_axis',(0.,-1.,0.)) ;
#9918=DIRECTION('ref_axis',(0.323867587734909,0.,-0.946102418142334)) ;
#9919=DIRECTION('center_axis',(2.86285518001772E-14,1.,9.80006109242406E-15)) ;
#9920=DIRECTION('ref_axis',(-0.323868053924072,1.34246448737236E-20,0.946102258557411)) ;
#9921=DIRECTION('center_axis',(0.,1.,0.)) ;
#9922=DIRECTION('ref_axis',(0.982473666441365,0.,-0.186401434407735)) ;
#9923=DIRECTION('center_axis',(5.20045044510935E-15,-1.,2.21184655932972E-14)) ;
#9924=DIRECTION('ref_axis',(0.98247394286439,9.86425565709368E-16,-0.186399977447689)) ;
#9925=DIRECTION('center_axis',(0.,-1.,0.)) ;
#9926=DIRECTION('ref_axis',(-0.51913214316201,0.,-0.854693990815437)) ;
#9927=DIRECTION('center_axis',(1.328521953279E-16,1.,5.52953428666426E-16)) ;
#9928=DIRECTION('ref_axis',(-0.0741867580339955,-5.55111512312574E-16,0.997244365706022)) ;
#9929=DIRECTION('',(0.,1.,0.)) ;
#9930=DIRECTION('center_axis',(0.,-1.,0.)) ;
#9931=DIRECTION('ref_axis',(-0.230203180796986,0.,0.973142587471615)) ;
#9932=DIRECTION('',(0.,-1.,0.)) ;
#9933=DIRECTION('',(1.55820775385987E-15,-1.,0.)) ;
#9934=DIRECTION('center_axis',(0.,1.,0.)) ;
#9935=DIRECTION('ref_axis',(-0.946102418141937,0.,-0.323867587736068)) ;
#9936=DIRECTION('',(0.,-1.,0.)) ;
#9937=DIRECTION('center_axis',(-2.45390046765461E-14,-1.,-8.40013522599915E-15)) ;
#9938=DIRECTION('ref_axis',(-0.910070204982191,2.58220234335356E-14,-0.414454125330746)) ;
#9939=DIRECTION('center_axis',(0.,-1.,0.)) ;
#9940=DIRECTION('ref_axis',(0.414454297733063,0.,-0.910070126468611)) ;
#9941=DIRECTION('',(0.,-1.,0.)) ;
#9942=DIRECTION('center_axis',(0.,-1.,0.)) ;
#9943=DIRECTION('ref_axis',(-0.946102402572802,0.,-0.323867633217603)) ;
#9944=DIRECTION('center_axis',(0.,-1.,0.)) ;
#9945=DIRECTION('ref_axis',(-0.99990130540252,0.,0.0140491798457023)) ;
#9946=DIRECTION('center_axis',(1.48618877891001E-16,1.,-4.98150096463128E-16)) ;
#9947=DIRECTION('ref_axis',(0.821909814783993,1.58603289232165E-16,0.569617640493816)) ;
#9948=DIRECTION('',(0.,1.,0.)) ;
#9949=DIRECTION('center_axis',(0.,-1.,0.)) ;
#9950=DIRECTION('ref_axis',(-0.186399383787626,0.,-0.982474055496426)) ;
#9951=DIRECTION('',(1.55820775385987E-15,-1.,0.)) ;
#9952=DIRECTION('',(0.,-1.,0.)) ;
#9953=DIRECTION('center_axis',(0.,-1.,0.)) ;
#9954=DIRECTION('ref_axis',(-0.935564561363999,0.,0.353155704356858)) ;
#9955=DIRECTION('',(0.,-1.,-6.23283101543948E-15)) ;
#9956=DIRECTION('center_axis',(0.,1.,0.)) ;
#9957=DIRECTION('ref_axis',(-0.186399467458827,0.,-0.982474039621946)) ;
#9958=DIRECTION('',(1.55820775385987E-15,-1.,0.)) ;
#9959=DIRECTION('center_axis',(2.06734131486432E-15,-1.,1.08965395694644E-14)) ;
#9960=DIRECTION('ref_axis',(-0.0140491798343041,-1.09830586184606E-14,-0.99990130540268)) ;
#9961=DIRECTION('center_axis',(0.,-1.,0.)) ;
#9962=DIRECTION('ref_axis',(0.99990130540221,0.,-0.0140491798677303)) ;
#9963=DIRECTION('center_axis',(0.,-1.,0.)) ;
#9964=DIRECTION('ref_axis',(-0.958437301458723,0.,0.285303240732594)) ;
#9965=DIRECTION('',(0.,1.,0.)) ;
#9966=DIRECTION('',(0.367081861009792,-0.707106776692743,0.604359920637352)) ;
#9967=DIRECTION('',(0.688115764120616,-0.707106780936084,0.162778056023868)) ;
#9968=DIRECTION('',(0.688115718421299,0.707106780933206,0.162778249222119)) ;
#9969=DIRECTION('',(0.643516818589292,-0.707106775388879,0.293063324883645)) ;
#9970=DIRECTION('',(-0.643516754494961,-0.707106778210615,-0.293063458815452)) ;
#9971=DIRECTION('',(0.707036994066234,-0.707106780687713,-0.00993427034270016)) ;
#9972=DIRECTION('',(-0.249719016897138,-0.707106780355147,-0.661543962088465)) ;
#9973=DIRECTION('',(-0.00993427042518335,-0.707106777296336,-0.707036997456787)) ;
#9974=DIRECTION('',(0.249718850397837,-0.707106779276632,0.661544026091243)) ;
#9975=DIRECTION('',(0.00993427042313984,-0.707106778684187,0.707036996068828)) ;
#9976=DIRECTION('',(0.677717522537246,-0.7071067736206,-0.201739858099097)) ;
#113314=CARTESIAN_POINT('Origin',(-8.09169626799648,-6.19999999995041,87.0702317281296)) ;
#113315=CARTESIAN_POINT('',(-23.3714287291853,-6.19999999995041,111.412782357318)) ;
#113316=CARTESIAN_POINT('',(-2.77488334235144,-6.19999999995041,115.314903713015)) ;
#113317=CARTESIAN_POINT('Origin',(-8.09169626799648,-6.19999999995041,87.0702317281297)) ;
#113318=CARTESIAN_POINT('',(-2.77488334235144,-9.1999999999504,115.314903713015)) ;
#113319=CARTESIAN_POINT('',(-2.77488334235144,-6.19999999995041,115.314903713015)) ;
#113320=CARTESIAN_POINT('',(-23.3714287291853,-9.1999999999504,111.412782357318)) ;
#113321=CARTESIAN_POINT('Origin',(-8.09169626799648,-9.19999999995042,87.0702317281297)) ;
#113322=CARTESIAN_POINT('',(-23.3714287291853,-6.19999999995041,111.412782357318)) ;
#113323=CARTESIAN_POINT('Origin',(-3.99680288865056E-14,-6.19999999995041,
130.056003483261)) ;
#113324=CARTESIAN_POINT('',(-11.2264641357303,-6.19999999995041,140.004194424792)) ;
#113325=CARTESIAN_POINT('Origin',(-8.32667268468867E-14,-6.19999999995041,
130.056003483261)) ;
#113326=CARTESIAN_POINT('',(-11.2264641357303,-9.1999999999504,140.004194424792)) ;
#113327=CARTESIAN_POINT('',(-11.2264641357303,-6.19999999995041,140.004194424792)) ;
#113328=CARTESIAN_POINT('Origin',(-8.32667268468867E-14,-9.1999999999504,
130.056003483261)) ;
#113329=CARTESIAN_POINT('Origin',(-32.7369214287718,-6.19999999995041,159.065417425019)) ;
#113330=CARTESIAN_POINT('',(-29.8935702991225,-6.19999999995041,130.4656735525)) ;
#113331=CARTESIAN_POINT('Origin',(-32.7369214287721,-6.19999999995039,159.06541742502)) ;
#113332=CARTESIAN_POINT('',(-29.8935702991225,-9.1999999999504,130.4656735525)) ;
#113333=CARTESIAN_POINT('',(-29.8935702991225,-6.19999999995041,130.4656735525)) ;
#113334=CARTESIAN_POINT('Origin',(-32.7369214287721,-9.19999999995039,159.06541742502)) ;
#113335=CARTESIAN_POINT('Origin',(-28.8703041205684,-6.19999999995041,120.173187866852)) ;
#113336=CARTESIAN_POINT('Origin',(-28.8703041205685,-6.19999999995041,120.173187866852)) ;
#113337=CARTESIAN_POINT('Origin',(-28.8703041205685,-9.1999999999504,120.173187866852)) ;
#113338=CARTESIAN_POINT('Origin',(-27.8320398342445,-6.19999999995041,121.882575848483)) ;
#113339=CARTESIAN_POINT('',(-27.8320398342445,-6.19999999995041,121.882575848483)) ;
#113340=CARTESIAN_POINT('Origin',(-28.8703041205685,-6.19999999995041,120.173187866852)) ;
#113341=CARTESIAN_POINT('',(-20.9452546314344,-6.19999999995041,120.517345819523)) ;
#113342=CARTESIAN_POINT('',(-22.3968662121113,-6.19999999995041,124.757884432279)) ;
#113343=CARTESIAN_POINT('Origin',(-4.52793358363124E-11,-6.19999999995017,
130.056003483244)) ;
#113344=CARTESIAN_POINT('',(-16.3949039990916,-6.19999999995041,122.589617308188)) ;
#113345=CARTESIAN_POINT('Origin',(-18.6700795113902,-6.19999999995041,121.553481994517)) ;
#113346=CARTESIAN_POINT('',(-17.5311532747538,-6.19999999995041,125.908900336264)) ;
#113347=CARTESIAN_POINT('Origin',(-5.38680211548126E-12,-6.19999999995041,
130.056003483259)) ;
#113348=CARTESIAN_POINT('Origin',(-19.9640098891907,-6.19999999995041,125.333393000438)) ;
#113349=CARTESIAN_POINT('',(6.99930913781763,-6.19999999995041,129.957659224341)) ;
#113350=CARTESIAN_POINT('Origin',(-1.22124532708767E-14,-6.19999999995041,
130.056003483261)) ;
#113351=CARTESIAN_POINT('',(-28.9640348151852,-6.19999999995041,113.502233048948)) ;
#113352=CARTESIAN_POINT('',(-29.0061823547883,-6.19999999995041,110.502529132742)) ;
#113353=CARTESIAN_POINT('Origin',(-28.9851085850295,-6.19999999995041,112.002381090846)) ;
#113354=CARTESIAN_POINT('',(-31.2264258318076,-6.19999999995041,113.931464218094)) ;
#113355=CARTESIAN_POINT('Origin',(-28.8703041205684,-6.19999999995041,120.173187866868)) ;
#113356=CARTESIAN_POINT('',(-32.2858929448779,-6.19999999995041,111.124770534002)) ;
#113357=CARTESIAN_POINT('Origin',(-31.7561588567387,-6.19999999995041,112.528117175379)) ;
#113358=CARTESIAN_POINT('Origin',(-28.8703041205686,-6.19999999995048,120.173187866852)) ;
#113359=CARTESIAN_POINT('',(-4.72036737313531,-6.19999999995041,119.695237805925)) ;
#113360=CARTESIAN_POINT('Origin',(-5.67880467459402,-6.19999999995041,119.980541046657)) ;
#113361=CARTESIAN_POINT('Origin',(-27.8320398342445,-9.1999999999504,121.882575848483)) ;
#113362=CARTESIAN_POINT('',(7.14929433383964,-9.19999999995041,129.955551847362)) ;
#113363=CARTESIAN_POINT('Ctrl Pts',(7.14929433383963,-9.1999999999504,129.955551847362)) ;
#113364=CARTESIAN_POINT('Ctrl Pts',(7.1370004751631,-9.19999999995042,129.057296456148)) ;
#113365=CARTESIAN_POINT('Ctrl Pts',(6.75374615451857,-9.1999999999504,127.19071738259)) ;
#113366=CARTESIAN_POINT('Ctrl Pts',(5.12518384136061,-9.1999999999504,124.784808129301)) ;
#113367=CARTESIAN_POINT('Ctrl Pts',(2.67435373485517,-9.19999999995041,
123.224310876368)) ;
#113368=CARTESIAN_POINT('Ctrl Pts',(-0.102837066898579,-9.19999999995041,
122.735357418181)) ;
#113369=CARTESIAN_POINT('Ctrl Pts',(-2.86529415935288,-9.19999999995041,
123.302148743622)) ;
#113370=CARTESIAN_POINT('Ctrl Pts',(-5.27116535713755,-9.1999999999504,
124.93087591456)) ;
#113371=CARTESIAN_POINT('Ctrl Pts',(-6.83175658899844,-9.19999999995038,
127.38161602962)) ;
#113372=CARTESIAN_POINT('Ctrl Pts',(-7.32060317086497,-9.19999999995042,
130.158872314311)) ;
#113373=CARTESIAN_POINT('Ctrl Pts',(-6.75388794178746,-9.19999999995039,
132.921250670983)) ;
#113374=CARTESIAN_POINT('Ctrl Pts',(-5.12509175131467,-9.1999999999504,
135.327253035705)) ;
#113375=CARTESIAN_POINT('Ctrl Pts',(-2.67441151797393,-9.1999999999504,
136.887664374679)) ;
#113376=CARTESIAN_POINT('Ctrl Pts',(0.102882667250271,-9.19999999995039,
137.376664884276)) ;
#113377=CARTESIAN_POINT('Ctrl Pts',(2.8652376417193,-9.19999999995039,136.809852443687)) ;
#113378=CARTESIAN_POINT('Ctrl Pts',(5.27125844026773,-9.19999999995041,
135.181128649693)) ;
#113379=CARTESIAN_POINT('Ctrl Pts',(6.83158159539024,-9.19999999995041,
132.73040390682)) ;
#113380=CARTESIAN_POINT('Ctrl Pts',(7.16224251088857,-9.19999999995039,
130.853800044315)) ;
#113381=CARTESIAN_POINT('Ctrl Pts',(7.14929433383963,-9.1999999999504,129.955551847362)) ;
#113382=CARTESIAN_POINT('',(-22.5428375993846,-9.1999999999504,124.72335395111)) ;
#113383=CARTESIAN_POINT('',(-17.3851818777868,-9.1999999999504,125.943430776449)) ;
#113384=CARTESIAN_POINT('Ctrl Pts',(-22.5428375993846,-9.1999999999504,
124.72335395111)) ;
#113385=CARTESIAN_POINT('Ctrl Pts',(-22.6228705779793,-9.19999999995041,
125.060835468167)) ;
#113386=CARTESIAN_POINT('Ctrl Pts',(-22.6481146793898,-9.19999999995039,
125.767699651254)) ;
#113387=CARTESIAN_POINT('Ctrl Pts',(-22.2776969349358,-9.19999999995041,
126.761819581242)) ;
#113388=CARTESIAN_POINT('Ctrl Pts',(-21.5548924132103,-9.19999999995038,
127.538488856445)) ;
#113389=CARTESIAN_POINT('Ctrl Pts',(-20.5899677472564,-9.19999999995041,
127.979442878113)) ;
#113390=CARTESIAN_POINT('Ctrl Pts',(-19.5297019368864,-9.19999999995041,
128.017567454019)) ;
#113391=CARTESIAN_POINT('Ctrl Pts',(-18.5355543800929,-9.1999999999504,
127.64705299455)) ;
#113392=CARTESIAN_POINT('Ctrl Pts',(-17.7589647755576,-9.19999999995041,
126.924264376153)) ;
#113393=CARTESIAN_POINT('Ctrl Pts',(-17.4648406712947,-9.1999999999504,
126.281024045295)) ;
#113394=CARTESIAN_POINT('Ctrl Pts',(-17.3851818776801,-9.1999999999504,
125.943430776462)) ;
#113395=CARTESIAN_POINT('',(-16.2583934662271,-9.19999999981371,122.651785427944)) ;
#113396=CARTESIAN_POINT('Origin',(-4.21641852199826,-9.1999999999504,128.612648863915)) ;
#113397=CARTESIAN_POINT('',(-21.081765150282,-9.1999999999504,120.455177671548)) ;
#113398=CARTESIAN_POINT('Ctrl Pts',(-16.2583934638605,-9.1999999999504,
122.651785429014)) ;
#113399=CARTESIAN_POINT('Ctrl Pts',(-16.1144636094565,-9.1999999999504,
122.336215974813)) ;
#113400=CARTESIAN_POINT('Ctrl Pts',(-15.9527012801464,-9.19999999995041,
121.647653807036)) ;
#113401=CARTESIAN_POINT('Ctrl Pts',(-16.123402898105,-9.1999999999504,120.600585547852)) ;
#113402=CARTESIAN_POINT('Ctrl Pts',(-16.6819725346811,-9.1999999999504,
119.698547154189)) ;
#113403=CARTESIAN_POINT('Ctrl Pts',(-17.5431302078255,-9.19999999995039,
119.078935764952)) ;
#113404=CARTESIAN_POINT('Ctrl Pts',(-18.5758949488641,-9.1999999999504,
118.836030266143)) ;
#113405=CARTESIAN_POINT('Ctrl Pts',(-19.6230096138486,-9.19999999995042,
119.006827682583)) ;
#113406=CARTESIAN_POINT('Ctrl Pts',(-20.524962978159,-9.19999999995041,
119.565396591838)) ;
#113407=CARTESIAN_POINT('Ctrl Pts',(-20.9381860344248,-9.19999999995041,
120.139425207325)) ;
#113408=CARTESIAN_POINT('Ctrl Pts',(-21.081765150282,-9.1999999999504,120.455177671548)) ;
#113409=CARTESIAN_POINT('Origin',(-5.46730600432587,-9.19999999995093,128.184444950592)) ;
#113410=CARTESIAN_POINT('',(-4.57660177482253,-9.19999999995041,119.652442318957)) ;
#113411=CARTESIAN_POINT('Ctrl Pts',(-4.57660177482253,-9.1999999999504,
119.652442318957)) ;
#113412=CARTESIAN_POINT('Ctrl Pts',(-4.66090400079055,-9.19999999995039,
119.363676940337)) ;
#113413=CARTESIAN_POINT('Ctrl Pts',(-5.07231914777193,-9.19999999995039,
118.859385893862)) ;
#113414=CARTESIAN_POINT('Ctrl Pts',(-6.04236399869572,-9.19999999995039,
118.758213536859)) ;
#113415=CARTESIAN_POINT('Ctrl Pts',(-6.80048159967586,-9.19999999995041,
119.373645566077)) ;
#113416=CARTESIAN_POINT('Ctrl Pts',(-6.90081901473353,-9.1999999999504,
120.344304696983)) ;
#113417=CARTESIAN_POINT('Ctrl Pts',(-6.28597182491173,-9.19999999995039,
121.102070939682)) ;
#113418=CARTESIAN_POINT('Ctrl Pts',(-5.31469869100537,-9.19999999995039,
121.202705829313)) ;
#113419=CARTESIAN_POINT('Ctrl Pts',(-4.55790335108104,-9.1999999999504,
120.587495567235)) ;
#113420=CARTESIAN_POINT('Ctrl Pts',(-4.48925688934139,-9.19999999995039,
119.940301972492)) ;
#113421=CARTESIAN_POINT('Ctrl Pts',(-4.57660177482253,-9.1999999999504,
119.652442318957)) ;
#113422=CARTESIAN_POINT('',(-29.0082897317938,-9.19999999985937,110.352543935372)) ;
#113423=CARTESIAN_POINT('',(-32.3388659738659,-9.1999999999504,110.984435725954)) ;
#113424=CARTESIAN_POINT('Origin',(-29.3248670281959,-9.1999999999504,117.777304321592)) ;
#113425=CARTESIAN_POINT('',(-31.1734524639126,-9.1999999999504,114.071798898544)) ;
#113426=CARTESIAN_POINT('Ctrl Pts',(-32.3388659738659,-9.1999999999504,
110.984435725954)) ;
#113427=CARTESIAN_POINT('Ctrl Pts',(-32.7450041950327,-9.1999999999504,
111.13470650637)) ;
#113428=CARTESIAN_POINT('Ctrl Pts',(-33.250393360795,-9.1999999999504,111.615093587184)) ;
#113429=CARTESIAN_POINT('Ctrl Pts',(-33.4478232528979,-9.1999999999504,
112.474879142272)) ;
#113430=CARTESIAN_POINT('Ctrl Pts',(-33.3403541520526,-9.1999999999504,
113.125956337085)) ;
#113431=CARTESIAN_POINT('Ctrl Pts',(-32.9905552298659,-9.19999999995041,
113.686234783214)) ;
#113432=CARTESIAN_POINT('Ctrl Pts',(-32.2744514960019,-9.1999999999504,
114.200426654396)) ;
#113433=CARTESIAN_POINT('Ctrl Pts',(-31.5775476849482,-9.1999999999504,
114.227645696731)) ;
#113434=CARTESIAN_POINT('Ctrl Pts',(-31.1734524639126,-9.1999999999504,
114.071798898544)) ;
#113435=CARTESIAN_POINT('',(-28.9619274381839,-9.19999999988973,113.652218245759)) ;
#113436=CARTESIAN_POINT('Origin',(-29.1721385651905,-9.1999999999503,118.58228377673)) ;
#113437=CARTESIAN_POINT('Ctrl Pts',(-28.9619274381555,-9.1999999999504,
113.652218246912)) ;
#113438=CARTESIAN_POINT('Ctrl Pts',(-28.5288930381478,-9.19999999995042,
113.648976325215)) ;
#113439=CARTESIAN_POINT('Ctrl Pts',(-27.8902872163334,-9.1999999999504,
113.369024853141)) ;
#113440=CARTESIAN_POINT('Ctrl Pts',(-27.4123099953964,-9.19999999995041,
112.627574967391)) ;
#113441=CARTESIAN_POINT('Ctrl Pts',(-27.2920262774471,-9.1999999999504,
111.978742812502)) ;
#113442=CARTESIAN_POINT('Ctrl Pts',(-27.4305073144874,-9.1999999999504,
111.332914318425)) ;
#113443=CARTESIAN_POINT('Ctrl Pts',(-27.9291423031889,-9.1999999999504,
110.605892050379)) ;
#113444=CARTESIAN_POINT('Ctrl Pts',(-28.5752805886998,-9.1999999999504,
110.343363232169)) ;
#113445=CARTESIAN_POINT('Ctrl Pts',(-29.0082897318249,-9.1999999999504,
110.352543933643)) ;
#113446=CARTESIAN_POINT('',(-27.7541700117984,-9.19999999995041,122.010779948746)) ;
#113447=CARTESIAN_POINT('Ctrl Pts',(-27.7541700117984,-9.1999999999504,
122.010779948746)) ;
#113448=CARTESIAN_POINT('Ctrl Pts',(-27.5135754621942,-9.19999999995041,
121.864832555746)) ;
#113449=CARTESIAN_POINT('Ctrl Pts',(-27.0907457483677,-9.19999999995038,
121.476859181283)) ;
#113450=CARTESIAN_POINT('Ctrl Pts',(-26.7272384292546,-9.1999999999504,
120.696662196726)) ;
#113451=CARTESIAN_POINT('Ctrl Pts',(-26.6900822991809,-9.1999999999504,
119.836671299616)) ;
#113452=CARTESIAN_POINT('Ctrl Pts',(-26.9848031252087,-9.19999999995041,
119.027970122367)) ;
#113453=CARTESIAN_POINT('Ctrl Pts',(-27.5665894666998,-9.1999999999504,
118.393586161041)) ;
#113454=CARTESIAN_POINT('Ctrl Pts',(-28.3468505140607,-9.19999999995041,
118.030145323177)) ;
#113455=CARTESIAN_POINT('Ctrl Pts',(-29.2068096659533,-9.19999999995039,
117.992953394567)) ;
#113456=CARTESIAN_POINT('Ctrl Pts',(-30.0155279148894,-9.19999999995041,
118.287693856939)) ;
#113457=CARTESIAN_POINT('Ctrl Pts',(-30.6499023447983,-9.1999999999504,
118.869469187485)) ;
#113458=CARTESIAN_POINT('Ctrl Pts',(-31.0133486320491,-9.1999999999504,
119.649736536709)) ;
#113459=CARTESIAN_POINT('Ctrl Pts',(-31.0505375041286,-9.1999999999504,
120.50969215252)) ;
#113460=CARTESIAN_POINT('Ctrl Pts',(-30.755798733008,-9.19999999995039,
121.318412358944)) ;
#113461=CARTESIAN_POINT('Ctrl Pts',(-30.1740208511346,-9.19999999995042,
121.95278610807)) ;
#113462=CARTESIAN_POINT('Ctrl Pts',(-29.3937430936942,-9.1999999999504,
122.316256382307)) ;
#113463=CARTESIAN_POINT('Ctrl Pts',(-28.5338133666822,-9.19999999995043,
122.353369994526)) ;
#113464=CARTESIAN_POINT('Ctrl Pts',(-27.9946120019688,-9.1999999999504,
122.1570111193)) ;
#113465=CARTESIAN_POINT('Ctrl Pts',(-27.7541700117984,-9.1999999999504,
122.010779948746)) ;
#113466=CARTESIAN_POINT('Origin',(-28.8703041205685,-6.19999999995041,120.173187866852)) ;
#113467=CARTESIAN_POINT('',(-27.8320398342445,-9.0499999999504,121.882575848483)) ;
#113468=CARTESIAN_POINT('Origin',(-28.8703041205684,-9.0499999999504,120.173187866852)) ;
#113469=CARTESIAN_POINT('',(-27.8320398342445,-6.19999999995041,121.882575848483)) ;
#113470=CARTESIAN_POINT('Origin',(-19.9640098891909,-6.19999999995041,125.333393000438)) ;
#113471=CARTESIAN_POINT('',(-22.3968662121113,-9.0499999999504,124.757884432279)) ;
#113472=CARTESIAN_POINT('',(-22.3968662121113,-6.19999999995041,124.757884432279)) ;
#113473=CARTESIAN_POINT('',(-17.5311532747538,-9.0499999999504,125.908900336264)) ;
#113474=CARTESIAN_POINT('',(-17.5311532747538,-6.19999999995041,125.908900336264)) ;
#113475=CARTESIAN_POINT('Ctrl Pts',(-22.3968662121113,-9.0499999999504,
124.757884432279)) ;
#113476=CARTESIAN_POINT('Ctrl Pts',(-22.4723690285854,-9.04999999995042,
125.076263256322)) ;
#113477=CARTESIAN_POINT('Ctrl Pts',(-22.4961842209104,-9.04999999995039,
125.743116253558)) ;
#113478=CARTESIAN_POINT('Ctrl Pts',(-22.1467335154594,-9.04999999995042,
126.680965246019)) ;
#113479=CARTESIAN_POINT('Ctrl Pts',(-21.4648424596514,-9.04999999995038,
127.4136721109)) ;
#113480=CARTESIAN_POINT('Ctrl Pts',(-20.5545361708193,-9.04999999995042,
127.829666467211)) ;
#113481=CARTESIAN_POINT('Ctrl Pts',(-19.5542854041389,-9.04999999995041,
127.865633052449)) ;
#113482=CARTESIAN_POINT('Ctrl Pts',(-18.6164103552122,-9.04999999995039,
127.516091106774)) ;
#113483=CARTESIAN_POINT('Ctrl Pts',(-17.8837786462394,-9.04999999995041,
126.834215051392)) ;
#113484=CARTESIAN_POINT('Ctrl Pts',(-17.6063030831261,-9.0499999999504,
126.227384554924)) ;
#113485=CARTESIAN_POINT('Ctrl Pts',(-17.5311532747538,-9.0499999999504,
125.908900336264)) ;
#113486=CARTESIAN_POINT('Origin',(-5.63105118089879E-12,-6.19999999995041,
130.056003483259)) ;
#113487=CARTESIAN_POINT('',(-16.3949039990916,-9.0499999999504,122.589617308188)) ;
#113488=CARTESIAN_POINT('',(-16.3949039990916,-6.19999999995041,122.589617308188)) ;
#113489=CARTESIAN_POINT('Origin',(-5.79536418854332E-12,-9.04999999995087,
130.056003483259)) ;
#113490=CARTESIAN_POINT('Origin',(-18.6700795113902,-6.19999999995041,121.553481994517)) ;
#113491=CARTESIAN_POINT('',(-20.9452546314344,-9.0499999999504,120.517345819523)) ;
#113492=CARTESIAN_POINT('',(-20.9452546314344,-6.19999999995041,120.517345819523)) ;
#113493=CARTESIAN_POINT('Ctrl Pts',(-16.3949039990916,-9.0499999999504,
122.589617308188)) ;
#113494=CARTESIAN_POINT('Ctrl Pts',(-16.2591211104845,-9.0499999999504,
122.291910279286)) ;
#113495=CARTESIAN_POINT('Ctrl Pts',(-16.1065151442268,-9.0499999999504,
121.642323325885)) ;
#113496=CARTESIAN_POINT('Ctrl Pts',(-16.2675544036708,-9.04999999995041,
120.654523083266)) ;
#113497=CARTESIAN_POINT('Ctrl Pts',(-16.7945068920798,-9.0499999999504,
119.803543465656)) ;
#113498=CARTESIAN_POINT('Ctrl Pts',(-17.6069197915061,-9.04999999995039,
119.219004419472)) ;
#113499=CARTESIAN_POINT('Ctrl Pts',(-18.5812261501238,-9.0499999999504,
118.989848288481)) ;
#113500=CARTESIAN_POINT('Ctrl Pts',(-19.5690701747728,-9.04999999995041,
119.150977926698)) ;
#113501=CARTESIAN_POINT('Ctrl Pts',(-20.419969573241,-9.04999999995041,
119.677929727982)) ;
#113502=CARTESIAN_POINT('Ctrl Pts',(-20.8098026478821,-9.04999999995041,
120.219466157043)) ;
#113503=CARTESIAN_POINT('Ctrl Pts',(-20.9452546314344,-9.0499999999504,
120.517345819523)) ;
#113504=CARTESIAN_POINT('Origin',(-4.50262049866978E-11,-6.19999999995041,
130.056003483244)) ;
#113505=CARTESIAN_POINT('Ctrl Pts',(-20.9452546314344,-9.0499999999504,
120.517345819523)) ;
#113506=CARTESIAN_POINT('Ctrl Pts',(-21.2554121720413,-9.04995061204382,
121.198398530804)) ;
#113507=CARTESIAN_POINT('Ctrl Pts',(-21.5321680097022,-9.05001239471631,
121.894174275922)) ;
#113508=CARTESIAN_POINT('Ctrl Pts',(-22.0169032426545,-9.05001239471625,
123.310213180309)) ;
#113509=CARTESIAN_POINT('Ctrl Pts',(-22.2245933795366,-9.04995061204343,
124.029631339807)) ;
#113510=CARTESIAN_POINT('Ctrl Pts',(-22.3968662121113,-9.04999999995041,
124.757884432279)) ;
#113511=CARTESIAN_POINT('Origin',(-3.33066907387547E-14,-6.19999999995041,
130.056003483261)) ;
#113512=CARTESIAN_POINT('',(6.99930913781763,-9.0499999999504,129.957659224341)) ;
#113513=CARTESIAN_POINT('Origin',(-8.88178419700125E-15,-9.0499999999504,
130.056003483261)) ;
#113514=CARTESIAN_POINT('',(6.99930913781758,-6.19999999995041,129.957659224341)) ;
#113515=CARTESIAN_POINT('Origin',(-28.8703041205686,-6.1999999999504,120.173187866852)) ;
#113516=CARTESIAN_POINT('',(-29.0061823547883,-9.0499999999504,110.502529132742)) ;
#113517=CARTESIAN_POINT('',(-29.0061823547883,-6.19999999995041,110.502529132742)) ;
#113518=CARTESIAN_POINT('',(-32.2858926954066,-9.04999999991833,111.124770439505)) ;
#113519=CARTESIAN_POINT('',(-32.2858929448779,-6.19999999995041,111.124770534002)) ;
#113520=CARTESIAN_POINT('Ctrl Pts',(-29.0061823547883,-9.04999999995044,
110.502529132742)) ;
#113521=CARTESIAN_POINT('Ctrl Pts',(-29.5656395665731,-9.04979411927751,
110.510389823533)) ;
#113522=CARTESIAN_POINT('Ctrl Pts',(-30.1233656337281,-9.05005210980387,
110.566783181888)) ;
#113523=CARTESIAN_POINT('Ctrl Pts',(-31.2228076802224,-9.0500521214643,
110.775374244021)) ;
#113524=CARTESIAN_POINT('Ctrl Pts',(-31.7624325937661,-9.04979414280626,
110.927175193771)) ;
#113525=CARTESIAN_POINT('Ctrl Pts',(-32.2858925706799,-9.04999999980325,
111.124770392751)) ;
#113526=CARTESIAN_POINT('Origin',(-31.7561588567387,-6.19999999995041,112.528117175379)) ;
#113527=CARTESIAN_POINT('',(-31.2264258318076,-9.0499999999504,113.931464218094)) ;
#113528=CARTESIAN_POINT('',(-31.2264258318076,-6.19999999995041,113.931464218094)) ;
#113529=CARTESIAN_POINT('Ctrl Pts',(-32.2858926956549,-9.0499999999504,
111.124770438834)) ;
#113530=CARTESIAN_POINT('Ctrl Pts',(-32.655109233656,-9.0499999999504,111.261380268983)) ;
#113531=CARTESIAN_POINT('Ctrl Pts',(-33.1145538702893,-9.04999999995041,
111.6980957759)) ;
#113532=CARTESIAN_POINT('Ctrl Pts',(-33.2940355805978,-9.0499999999504,
112.479718963136)) ;
#113533=CARTESIAN_POINT('Ctrl Pts',(-33.1963363978295,-9.0499999999504,
113.071607322719)) ;
#113534=CARTESIAN_POINT('Ctrl Pts',(-32.878337377691,-9.04999999995041,
113.580951364404)) ;
#113535=CARTESIAN_POINT('Ctrl Pts',(-32.2273339833429,-9.04999999995041,
114.048398519428)) ;
#113536=CARTESIAN_POINT('Ctrl Pts',(-31.5937850640421,-9.0499999999504,
114.073143104941)) ;
#113537=CARTESIAN_POINT('Ctrl Pts',(-31.2264258318076,-9.0499999999504,
113.931464218094)) ;
#113538=CARTESIAN_POINT('Origin',(-28.8703041205683,-6.19999999995041,120.173187866869)) ;
#113539=CARTESIAN_POINT('',(-28.9640348151852,-9.0499999999504,113.502233048948)) ;
#113540=CARTESIAN_POINT('',(-28.9640348151852,-6.19999999995041,113.502233048948)) ;
#113541=CARTESIAN_POINT('Origin',(-28.8703041205685,-9.04999999995033,120.173187866868)) ;
#113542=CARTESIAN_POINT('Origin',(-28.9851085850296,-6.19999999995041,112.002381090846)) ;
#113543=CARTESIAN_POINT('Ctrl Pts',(-28.9640348151852,-9.0499999999504,
113.502233048948)) ;
#113544=CARTESIAN_POINT('Ctrl Pts',(-28.5703671785535,-9.04999999995041,
113.49928585092)) ;
#113545=CARTESIAN_POINT('Ctrl Pts',(-27.9898164318432,-9.0499999999504,
113.244784510051)) ;
#113546=CARTESIAN_POINT('Ctrl Pts',(-27.5552916853933,-9.0499999999504,
112.570739161072)) ;
#113547=CARTESIAN_POINT('Ctrl Pts',(-27.4459428508496,-9.0499999999504,
111.980891746487)) ;
#113548=CARTESIAN_POINT('Ctrl Pts',(-27.5718347027607,-9.04999999995039,
111.393774933819)) ;
#113549=CARTESIAN_POINT('Ctrl Pts',(-28.0251392380631,-9.04999999995041,
110.732845600627)) ;
#113550=CARTESIAN_POINT('Ctrl Pts',(-28.612537679088,-9.0499999999504,110.494183035205)) ;
#113551=CARTESIAN_POINT('Ctrl Pts',(-29.0061823547883,-9.0499999999504,
110.502529132742)) ;
#113552=CARTESIAN_POINT('Origin',(-5.67880467459403,-6.19999999995041,119.980541046657)) ;
#113553=CARTESIAN_POINT('',(-4.72036737313531,-9.0499999999504,119.695237805925)) ;
#113554=CARTESIAN_POINT('Ctrl Pts',(-4.72036737313531,-9.0499999999504,
119.695237805925)) ;
#113555=CARTESIAN_POINT('Ctrl Pts',(-4.79367365129389,-9.04999999995039,
119.444137474753)) ;
#113556=CARTESIAN_POINT('Ctrl Pts',(-5.15142595671263,-9.04999999995038,
119.005623523177)) ;
#113557=CARTESIAN_POINT('Ctrl Pts',(-5.99494321694567,-9.04999999995039,
118.917647559852)) ;
#113558=CARTESIAN_POINT('Ctrl Pts',(-6.65417591390635,-9.04999999995041,
119.452805846097)) ;
#113559=CARTESIAN_POINT('Ctrl Pts',(-6.74142583978821,-9.0499999999504,
120.296857264431)) ;
#113560=CARTESIAN_POINT('Ctrl Pts',(-6.2067761094534,-9.04999999995039,
120.955784431796)) ;
#113561=CARTESIAN_POINT('Ctrl Pts',(-5.36219077623412,-9.04999999995039,
121.043293031702)) ;
#113562=CARTESIAN_POINT('Ctrl Pts',(-4.70410787109404,-9.04999999995041,
120.508327585707)) ;
#113563=CARTESIAN_POINT('Ctrl Pts',(-4.64441529656359,-9.0499999999504,
119.945550548028)) ;
#113564=CARTESIAN_POINT('Ctrl Pts',(-4.72036737313531,-9.0499999999504,
119.695237805925)) ;
#113565=CARTESIAN_POINT('',(-4.72036737313532,-6.19999999995041,119.695237805925)) ;
#113566=CARTESIAN_POINT('Ctrl Pts',(-27.8361237168375,-9.04213325042268,
121.875852184848)) ;
#113567=CARTESIAN_POINT('Ctrl Pts',(-27.7541700117984,-9.1999999999504,
122.010779948746)) ;
#113568=CARTESIAN_POINT('Ctrl Pts',(-27.6131951563421,-9.04213325042269,
121.740621185333)) ;
#113569=CARTESIAN_POINT('Ctrl Pts',(-27.5135754621942,-9.19999999995041,
121.864832555746)) ;
#113570=CARTESIAN_POINT('Ctrl Pts',(-27.2214123048267,-9.04213325042267,
121.381135295391)) ;
#113571=CARTESIAN_POINT('Ctrl Pts',(-27.0907457483677,-9.19999999995038,
121.476859181283)) ;
#113572=CARTESIAN_POINT('Ctrl Pts',(-26.8845960173112,-9.04213325042268,
120.658225363553)) ;
#113573=CARTESIAN_POINT('Ctrl Pts',(-26.7272384292546,-9.1999999999504,
120.696662196726)) ;
#113574=CARTESIAN_POINT('Ctrl Pts',(-26.8501681278626,-9.04213325042268,
119.861380498453)) ;
#113575=CARTESIAN_POINT('Ctrl Pts',(-26.6900822991809,-9.1999999999504,
119.836671299616)) ;
#113576=CARTESIAN_POINT('Ctrl Pts',(-27.1232486667411,-9.04213325042269,
119.112059332406)) ;
#113577=CARTESIAN_POINT('Ctrl Pts',(-26.9848031252087,-9.19999999995041,
119.027970122367)) ;
#113578=CARTESIAN_POINT('Ctrl Pts',(-27.6623165339235,-9.04213325042267,
118.524255899387)) ;
#113579=CARTESIAN_POINT('Ctrl Pts',(-27.5665894666998,-9.1999999999504,
118.393586161041)) ;
#113580=CARTESIAN_POINT('Ctrl Pts',(-28.3852858260732,-9.04213325042269,
118.187501211538)) ;
#113581=CARTESIAN_POINT('Ctrl Pts',(-28.3468505140607,-9.19999999995041,
118.030145323177)) ;
#113582=CARTESIAN_POINT('Ctrl Pts',(-29.182101276225,-9.04213325042267,
118.15304015244)) ;
#113583=CARTESIAN_POINT('Ctrl Pts',(-29.2068096659533,-9.19999999995039,
117.992953394567)) ;
#113584=CARTESIAN_POINT('Ctrl Pts',(-29.9314382607409,-9.04213325042269,
118.426138885432)) ;
#113585=CARTESIAN_POINT('Ctrl Pts',(-30.0155279148894,-9.19999999995041,
118.287693856939)) ;
#113586=CARTESIAN_POINT('Ctrl Pts',(-30.5192328620952,-9.04213325042268,
118.965196550334)) ;
#113587=CARTESIAN_POINT('Ctrl Pts',(-30.6499023447983,-9.1999999999504,
118.869469187485)) ;
#113588=CARTESIAN_POINT('Ctrl Pts',(-30.8559925991121,-9.04213325042268,
119.688171680639)) ;
#113589=CARTESIAN_POINT('Ctrl Pts',(-31.0133486320491,-9.1999999999504,
119.649736536709)) ;
#113590=CARTESIAN_POINT('Ctrl Pts',(-30.8904508259688,-9.04213325042268,
120.484983855758)) ;
#113591=CARTESIAN_POINT('Ctrl Pts',(-31.0505375041286,-9.1999999999504,
120.50969215252)) ;
#113592=CARTESIAN_POINT('Ctrl Pts',(-30.61735366085,-9.04213325042268,121.23432265262)) ;
#113593=CARTESIAN_POINT('Ctrl Pts',(-30.755798733008,-9.19999999995039,
121.318412358944)) ;
#113594=CARTESIAN_POINT('Ctrl Pts',(-30.0782936311612,-9.04213325042269,
121.82211662443)) ;
#113595=CARTESIAN_POINT('Ctrl Pts',(-30.1740208511346,-9.19999999995042,
121.95278610807)) ;
#113596=CARTESIAN_POINT('Ctrl Pts',(-29.3553088569288,-9.04213325042268,
122.158898586878)) ;
#113597=CARTESIAN_POINT('Ctrl Pts',(-29.3937430936942,-9.1999999999504,
122.316256382307)) ;
#113598=CARTESIAN_POINT('Ctrl Pts',(-28.5585206705951,-9.0421332504227,
122.193287079418)) ;
#113599=CARTESIAN_POINT('Ctrl Pts',(-28.5338133666822,-9.19999999995043,
122.353369994526)) ;
#113600=CARTESIAN_POINT('Ctrl Pts',(-28.0589109164076,-9.04213325042268,
122.011346130603)) ;
#113601=CARTESIAN_POINT('Ctrl Pts',(-27.9946120019688,-9.1999999999504,
122.1570111193)) ;
#113602=CARTESIAN_POINT('Ctrl Pts',(-27.8361237168375,-9.04213325042268,
121.875852184848)) ;
#113603=CARTESIAN_POINT('Ctrl Pts',(-27.7541700117984,-9.1999999999504,
122.010779948746)) ;
#113604=CARTESIAN_POINT('',(-27.8320398342445,-9.0499999999504,121.882575848483)) ;
#113605=CARTESIAN_POINT('Ctrl Pts',(-22.3968662121113,-9.0499999999504,
124.757884432279)) ;
#113606=CARTESIAN_POINT('Ctrl Pts',(-22.5428375993846,-9.1999999999504,
124.72335395111)) ;
#113607=CARTESIAN_POINT('Ctrl Pts',(-22.4723690285854,-9.04999999995042,
125.076263256322)) ;
#113608=CARTESIAN_POINT('Ctrl Pts',(-22.6228705779793,-9.19999999995041,
125.060835468167)) ;
#113609=CARTESIAN_POINT('Ctrl Pts',(-22.4961842209104,-9.04999999995039,
125.743116253558)) ;
#113610=CARTESIAN_POINT('Ctrl Pts',(-22.6481146793898,-9.19999999995039,
125.767699651254)) ;
#113611=CARTESIAN_POINT('Ctrl Pts',(-22.1467335154594,-9.04999999995042,
126.680965246019)) ;
#113612=CARTESIAN_POINT('Ctrl Pts',(-22.2776969349358,-9.19999999995041,
126.761819581242)) ;
#113613=CARTESIAN_POINT('Ctrl Pts',(-21.4648424596514,-9.04999999995038,
127.4136721109)) ;
#113614=CARTESIAN_POINT('Ctrl Pts',(-21.5548924132103,-9.19999999995038,
127.538488856445)) ;
#113615=CARTESIAN_POINT('Ctrl Pts',(-20.5545361708193,-9.04999999995042,
127.829666467211)) ;
#113616=CARTESIAN_POINT('Ctrl Pts',(-20.5899677472564,-9.19999999995041,
127.979442878113)) ;
#113617=CARTESIAN_POINT('Ctrl Pts',(-19.5542854041389,-9.04999999995041,
127.865633052449)) ;
#113618=CARTESIAN_POINT('Ctrl Pts',(-19.5297019368864,-9.19999999995041,
128.017567454019)) ;
#113619=CARTESIAN_POINT('Ctrl Pts',(-18.6164103552122,-9.04999999995039,
127.516091106774)) ;
#113620=CARTESIAN_POINT('Ctrl Pts',(-18.5355543800929,-9.1999999999504,
127.64705299455)) ;
#113621=CARTESIAN_POINT('Ctrl Pts',(-17.8837786462394,-9.04999999995041,
126.834215051392)) ;
#113622=CARTESIAN_POINT('Ctrl Pts',(-17.7589647755576,-9.19999999995041,
126.924264376153)) ;
#113623=CARTESIAN_POINT('Ctrl Pts',(-17.6063030831261,-9.0499999999504,
126.227384554924)) ;
#113624=CARTESIAN_POINT('Ctrl Pts',(-17.4648406712947,-9.1999999999504,
126.281024045295)) ;
#113625=CARTESIAN_POINT('Ctrl Pts',(-17.5311532747538,-9.0499999999504,
125.908900336264)) ;
#113626=CARTESIAN_POINT('Ctrl Pts',(-17.3851818776801,-9.1999999999504,
125.943430776462)) ;
#113627=CARTESIAN_POINT('',(-17.5311532747538,-9.0499999999504,125.908900336264)) ;
#113628=CARTESIAN_POINT('',(-22.5428375993846,-9.1999999999504,124.72335395111)) ;
#113629=CARTESIAN_POINT('Ctrl Pts',(-17.5311532747538,-9.0499999999504,
125.908900336264)) ;
#113630=CARTESIAN_POINT('Ctrl Pts',(-17.3851818778934,-9.1999999999504,
125.943430776435)) ;
#113631=CARTESIAN_POINT('Ctrl Pts',(-17.2615869582204,-9.0499999999504,
124.769020077632)) ;
#113632=CARTESIAN_POINT('Ctrl Pts',(-17.1178600783809,-9.19999999995041,
124.813041616962)) ;
#113633=CARTESIAN_POINT('Ctrl Pts',(-16.8804331897069,-9.04999999995041,
123.655569656133)) ;
#113634=CARTESIAN_POINT('Ctrl Pts',(-16.7398799486353,-9.1999999999504,
123.708862229139)) ;
#113635=CARTESIAN_POINT('Ctrl Pts',(-16.3949039990916,-9.0499999999504,
122.589617308188)) ;
#113636=CARTESIAN_POINT('Ctrl Pts',(-16.2583934683448,-9.1999999999504,
122.651785426988)) ;
#113637=CARTESIAN_POINT('',(-16.3949039990916,-9.0499999999504,122.589617308188)) ;
#113638=CARTESIAN_POINT('Ctrl Pts',(-16.3949039990916,-9.0499999999504,
122.589617308188)) ;
#113639=CARTESIAN_POINT('Ctrl Pts',(-16.2583934638605,-9.1999999999504,
122.651785429014)) ;
#113640=CARTESIAN_POINT('Ctrl Pts',(-16.2591211104845,-9.0499999999504,
122.291910279286)) ;
#113641=CARTESIAN_POINT('Ctrl Pts',(-16.1144636094565,-9.1999999999504,
122.336215974813)) ;
#113642=CARTESIAN_POINT('Ctrl Pts',(-16.1065151442268,-9.0499999999504,
121.642323325885)) ;
#113643=CARTESIAN_POINT('Ctrl Pts',(-15.9527012801464,-9.19999999995041,
121.647653807036)) ;
#113644=CARTESIAN_POINT('Ctrl Pts',(-16.2675544036708,-9.04999999995041,
120.654523083266)) ;
#113645=CARTESIAN_POINT('Ctrl Pts',(-16.123402898105,-9.1999999999504,120.600585547852)) ;
#113646=CARTESIAN_POINT('Ctrl Pts',(-16.7945068920798,-9.0499999999504,
119.803543465656)) ;
#113647=CARTESIAN_POINT('Ctrl Pts',(-16.6819725346811,-9.1999999999504,
119.698547154189)) ;
#113648=CARTESIAN_POINT('Ctrl Pts',(-17.6069197915061,-9.04999999995039,
119.219004419472)) ;
#113649=CARTESIAN_POINT('Ctrl Pts',(-17.5431302078255,-9.19999999995039,
119.078935764952)) ;
#113650=CARTESIAN_POINT('Ctrl Pts',(-18.5812261501238,-9.0499999999504,
118.989848288481)) ;
#113651=CARTESIAN_POINT('Ctrl Pts',(-18.5758949488641,-9.1999999999504,
118.836030266143)) ;
#113652=CARTESIAN_POINT('Ctrl Pts',(-19.5690701747728,-9.04999999995041,
119.150977926698)) ;
#113653=CARTESIAN_POINT('Ctrl Pts',(-19.6230096138486,-9.19999999995042,
119.006827682583)) ;
#113654=CARTESIAN_POINT('Ctrl Pts',(-20.419969573241,-9.04999999995041,
119.677929727982)) ;
#113655=CARTESIAN_POINT('Ctrl Pts',(-20.524962978159,-9.19999999995041,
119.565396591838)) ;
#113656=CARTESIAN_POINT('Ctrl Pts',(-20.8098026478821,-9.04999999995041,
120.219466157043)) ;
#113657=CARTESIAN_POINT('Ctrl Pts',(-20.9381860344248,-9.19999999995041,
120.139425207325)) ;
#113658=CARTESIAN_POINT('Ctrl Pts',(-20.9452546314344,-9.0499999999504,
120.517345819523)) ;
#113659=CARTESIAN_POINT('Ctrl Pts',(-21.081765150282,-9.1999999999504,120.455177671548)) ;
#113660=CARTESIAN_POINT('',(-20.9452546314344,-9.0499999999504,120.517345819523)) ;
#113661=CARTESIAN_POINT('Ctrl Pts',(-20.9452096849757,-9.04995061204342,
120.517366288554)) ;
#113662=CARTESIAN_POINT('Ctrl Pts',(-21.081765150282,-9.1999999999504,120.455177671548)) ;
#113663=CARTESIAN_POINT('Ctrl Pts',(-21.5654945670341,-9.04995061204342,
121.879167117613)) ;
#113664=CARTESIAN_POINT('Ctrl Pts',(-21.706094083138,-9.1999999999504,121.825856991404)) ;
#113665=CARTESIAN_POINT('Ctrl Pts',(-22.0524352836959,-9.04995061204342,
123.301648819064)) ;
#113666=CARTESIAN_POINT('Ctrl Pts',(-22.1962094837586,-9.1999999999504,
123.257612778353)) ;
#113667=CARTESIAN_POINT('Ctrl Pts',(-22.396818150636,-9.04995061204342,
124.757895801533)) ;
#113668=CARTESIAN_POINT('Ctrl Pts',(-22.5428375993846,-9.1999999999504,
124.72335395111)) ;
#113669=CARTESIAN_POINT('Ctrl Pts',(6.98431061821543,-9.0349999999504,129.957869962039)) ;
#113670=CARTESIAN_POINT('Ctrl Pts',(7.14929433383963,-9.1999999999504,129.955551847362)) ;
#113671=CARTESIAN_POINT('Ctrl Pts',(6.97230046451942,-9.03499999995042,
129.080343541437)) ;
#113672=CARTESIAN_POINT('Ctrl Pts',(7.1370004751631,-9.19999999995042,129.057296456148)) ;
#113673=CARTESIAN_POINT('Ctrl Pts',(6.59789047376578,-9.0349999999504,127.256839369418)) ;
#113674=CARTESIAN_POINT('Ctrl Pts',(6.75374615451857,-9.1999999999504,127.19071738259)) ;
#113675=CARTESIAN_POINT('Ctrl Pts',(5.00691036833316,-9.03499999995039,
124.90645109918)) ;
#113676=CARTESIAN_POINT('Ctrl Pts',(5.12518384136061,-9.1999999999504,124.784808129301)) ;
#113677=CARTESIAN_POINT('Ctrl Pts',(2.61263787931452,-9.03499999995041,
123.381965321084)) ;
#113678=CARTESIAN_POINT('Ctrl Pts',(2.67435373485517,-9.19999999995041,
123.224310876368)) ;
#113679=CARTESIAN_POINT('Ctrl Pts',(-0.100463903727752,-9.0349999999504,
122.904295404302)) ;
#113680=CARTESIAN_POINT('Ctrl Pts',(-0.102837066898579,-9.19999999995041,
122.735357418181)) ;
#113681=CARTESIAN_POINT('Ctrl Pts',(-2.7991719865524,-9.0349999999504,123.458006929968)) ;
#113682=CARTESIAN_POINT('Ctrl Pts',(-2.86529415935288,-9.19999999995041,
123.302148743622)) ;
#113683=CARTESIAN_POINT('Ctrl Pts',(-5.14952307947999,-9.03499999995039,
125.049148089099)) ;
#113684=CARTESIAN_POINT('Ctrl Pts',(-5.27116535713755,-9.1999999999504,
124.93087591456)) ;
#113685=CARTESIAN_POINT('Ctrl Pts',(-6.67410066780377,-9.03499999995039,
127.443332663221)) ;
#113686=CARTESIAN_POINT('Ctrl Pts',(-6.83175658899844,-9.19999999995038,
127.38161602962)) ;
#113687=CARTESIAN_POINT('Ctrl Pts',(-7.15166617454153,-9.03499999995041,
130.156498418203)) ;
#113688=CARTESIAN_POINT('Ctrl Pts',(-7.32060317086497,-9.19999999995042,
130.158872314311)) ;
#113689=CARTESIAN_POINT('Ctrl Pts',(-6.59802898938665,-9.03499999995039,
132.855129581994)) ;
#113690=CARTESIAN_POINT('Ctrl Pts',(-6.75388794178746,-9.19999999995039,
132.921250670983)) ;
#113691=CARTESIAN_POINT('Ctrl Pts',(-5.00682040300008,-9.0349999999504,
135.2056088154)) ;
#113692=CARTESIAN_POINT('Ctrl Pts',(-5.12509175131467,-9.1999999999504,
135.327253035705)) ;
#113693=CARTESIAN_POINT('Ctrl Pts',(-2.61269432921154,-9.0349999999504,
136.730010661744)) ;
#113694=CARTESIAN_POINT('Ctrl Pts',(-2.67441151797393,-9.1999999999504,
136.887664374679)) ;
#113695=CARTESIAN_POINT('Ctrl Pts',(0.100508451930804,-9.03499999995039,
137.207726544253)) ;
#113696=CARTESIAN_POINT('Ctrl Pts',(0.102882667250271,-9.19999999995039,
137.376664884276)) ;
#113697=CARTESIAN_POINT('Ctrl Pts',(2.79911677297535,-9.0349999999504,136.653994390812)) ;
#113698=CARTESIAN_POINT('Ctrl Pts',(2.8652376417193,-9.19999999995039,136.809852443687)) ;
#113699=CARTESIAN_POINT('Ctrl Pts',(5.14961401488543,-9.03499999995041,
135.062856530293)) ;
#113700=CARTESIAN_POINT('Ctrl Pts',(5.27125844026773,-9.19999999995041,
135.181128649693)) ;
#113701=CARTESIAN_POINT('Ctrl Pts',(6.67392971230693,-9.0349999999504,132.668686974082)) ;
#113702=CARTESIAN_POINT('Ctrl Pts',(6.83158159539024,-9.19999999995041,
132.73040390682)) ;
#113703=CARTESIAN_POINT('Ctrl Pts',(6.99695999145945,-9.0349999999504,130.835389354393)) ;
#113704=CARTESIAN_POINT('Ctrl Pts',(7.16224251088857,-9.19999999995039,
130.853800044315)) ;
#113705=CARTESIAN_POINT('Ctrl Pts',(6.98431061821543,-9.0349999999504,129.957869962039)) ;
#113706=CARTESIAN_POINT('Ctrl Pts',(7.14929433383963,-9.1999999999504,129.955551847362)) ;
#113707=CARTESIAN_POINT('',(6.99930913781763,-9.0499999999504,129.957659224341)) ;
#113708=CARTESIAN_POINT('Ctrl Pts',(-29.0061794623337,-9.04979411927748,
110.502734993095)) ;
#113709=CARTESIAN_POINT('Ctrl Pts',(-29.0082897317652,-9.1999999999504,
110.35254393692)) ;
#113710=CARTESIAN_POINT('Ctrl Pts',(-30.1244489973375,-9.04979411927748,
110.518035751111)) ;
#113711=CARTESIAN_POINT('Ctrl Pts',(-30.1439270242023,-9.19999999995041,
110.368082329788)) ;
#113712=CARTESIAN_POINT('Ctrl Pts',(-31.2396537334849,-9.04979411927748,
110.729617347937)) ;
#113713=CARTESIAN_POINT('Ctrl Pts',(-31.2764519194819,-9.1999999999504,
110.582949984148)) ;
#113714=CARTESIAN_POINT('Ctrl Pts',(-32.2858198627326,-9.04979411927748,
111.12496300725)) ;
#113715=CARTESIAN_POINT('Ctrl Pts',(-32.3388659738659,-9.1999999999504,
110.984435725954)) ;
#113716=CARTESIAN_POINT('',(-32.2858925707319,-9.0499999999504,111.124770392613)) ;
#113717=CARTESIAN_POINT('',(-29.0061823547883,-9.0499999999504,110.502529132742)) ;
#113718=CARTESIAN_POINT('Ctrl Pts',(-32.2858925707319,-9.0499999999504,
111.124770392613)) ;
#113719=CARTESIAN_POINT('Ctrl Pts',(-32.3388659738659,-9.1999999999504,
110.984435725954)) ;
#113720=CARTESIAN_POINT('Ctrl Pts',(-32.6551091645665,-9.0499999999504,
111.261380203311)) ;
#113721=CARTESIAN_POINT('Ctrl Pts',(-32.7450041950327,-9.1999999999504,
111.13470650637)) ;
#113722=CARTESIAN_POINT('Ctrl Pts',(-33.1145538601681,-9.04999999995041,
111.698095731824)) ;
#113723=CARTESIAN_POINT('Ctrl Pts',(-33.250393360795,-9.1999999999504,111.615093587184)) ;
#113724=CARTESIAN_POINT('Ctrl Pts',(-33.2940355805978,-9.0499999999504,
112.479718963136)) ;
#113725=CARTESIAN_POINT('Ctrl Pts',(-33.4478232528979,-9.1999999999504,
112.474879142272)) ;
#113726=CARTESIAN_POINT('Ctrl Pts',(-33.1963363978295,-9.0499999999504,
113.071607322719)) ;
#113727=CARTESIAN_POINT('Ctrl Pts',(-33.3403541520526,-9.1999999999504,
113.125956337085)) ;
#113728=CARTESIAN_POINT('Ctrl Pts',(-32.878337377691,-9.04999999995041,
113.580951364404)) ;
#113729=CARTESIAN_POINT('Ctrl Pts',(-32.9905552298659,-9.19999999995041,
113.686234783214)) ;
#113730=CARTESIAN_POINT('Ctrl Pts',(-32.2273339833429,-9.04999999995041,
114.048398519428)) ;
#113731=CARTESIAN_POINT('Ctrl Pts',(-32.2744514960019,-9.1999999999504,
114.200426654396)) ;
#113732=CARTESIAN_POINT('Ctrl Pts',(-31.5937850640421,-9.0499999999504,
114.073143104941)) ;
#113733=CARTESIAN_POINT('Ctrl Pts',(-31.5775476849482,-9.1999999999504,
114.227645696731)) ;
#113734=CARTESIAN_POINT('Ctrl Pts',(-31.2264258318076,-9.0499999999504,
113.931464218094)) ;
#113735=CARTESIAN_POINT('Ctrl Pts',(-31.1734524639126,-9.1999999999504,
114.071798898544)) ;
#113736=CARTESIAN_POINT('',(-31.2264258318076,-9.0499999999504,113.931464218094)) ;
#113737=CARTESIAN_POINT('Ctrl Pts',(-31.2264258318076,-9.0499999999504,
113.931464218094)) ;
#113738=CARTESIAN_POINT('Ctrl Pts',(-31.1734524639126,-9.19999999995041,
114.071798898544)) ;
#113739=CARTESIAN_POINT('Ctrl Pts',(-30.5047503325303,-9.0499999999504,
113.658743196313)) ;
#113740=CARTESIAN_POINT('Ctrl Pts',(-30.4680025594377,-9.1999999999504,
113.805209524826)) ;
#113741=CARTESIAN_POINT('Ctrl Pts',(-29.7354496684938,-9.04999999995041,
113.512787956471)) ;
#113742=CARTESIAN_POINT('Ctrl Pts',(-29.7159983261929,-9.19999999995042,
113.662535842927)) ;
#113743=CARTESIAN_POINT('Ctrl Pts',(-28.9640348151852,-9.0499999999504,
113.502233048948)) ;
#113744=CARTESIAN_POINT('Ctrl Pts',(-28.9619274382105,-9.1999999999504,
113.652218244728)) ;
#113745=CARTESIAN_POINT('',(-28.9640348151852,-9.0499999999504,113.502233048948)) ;
#113746=CARTESIAN_POINT('Ctrl Pts',(-28.9640348151852,-9.0499999999504,
113.502233048948)) ;
#113747=CARTESIAN_POINT('Ctrl Pts',(-28.9619274381555,-9.1999999999504,
113.652218246912)) ;
#113748=CARTESIAN_POINT('Ctrl Pts',(-28.5703671785535,-9.04999999995041,
113.49928585092)) ;
#113749=CARTESIAN_POINT('Ctrl Pts',(-28.5288930381478,-9.19999999995042,
113.648976325215)) ;
#113750=CARTESIAN_POINT('Ctrl Pts',(-27.9898164318432,-9.0499999999504,
113.244784510051)) ;
#113751=CARTESIAN_POINT('Ctrl Pts',(-27.8902872163334,-9.1999999999504,
113.369024853141)) ;
#113752=CARTESIAN_POINT('Ctrl Pts',(-27.5552916853933,-9.0499999999504,
112.570739161072)) ;
#113753=CARTESIAN_POINT('Ctrl Pts',(-27.4123099953964,-9.19999999995041,
112.627574967391)) ;
#113754=CARTESIAN_POINT('Ctrl Pts',(-27.4459428508496,-9.0499999999504,
111.980891746487)) ;
#113755=CARTESIAN_POINT('Ctrl Pts',(-27.2920262774471,-9.1999999999504,
111.978742812502)) ;
#113756=CARTESIAN_POINT('Ctrl Pts',(-27.5718347027607,-9.04999999995039,
111.393774933819)) ;
#113757=CARTESIAN_POINT('Ctrl Pts',(-27.4305073144874,-9.1999999999504,
111.332914318425)) ;
#113758=CARTESIAN_POINT('Ctrl Pts',(-28.0251392380631,-9.04999999995041,
110.732845600627)) ;
#113759=CARTESIAN_POINT('Ctrl Pts',(-27.9291423031889,-9.1999999999504,
110.605892050379)) ;
#113760=CARTESIAN_POINT('Ctrl Pts',(-28.612537679088,-9.0499999999504,110.494183035205)) ;
#113761=CARTESIAN_POINT('Ctrl Pts',(-28.5752805886998,-9.1999999999504,
110.343363232169)) ;
#113762=CARTESIAN_POINT('Ctrl Pts',(-29.0061823547883,-9.0499999999504,
110.502529132742)) ;
#113763=CARTESIAN_POINT('Ctrl Pts',(-29.0082897318249,-9.1999999999504,
110.352543933643)) ;
#113764=CARTESIAN_POINT('Ctrl Pts',(-4.72036737313531,-9.0499999999504,
119.695237805925)) ;
#113765=CARTESIAN_POINT('Ctrl Pts',(-4.57660177482253,-9.1999999999504,
119.652442318957)) ;
#113766=CARTESIAN_POINT('Ctrl Pts',(-4.79367365129389,-9.04999999995039,
119.444137474753)) ;
#113767=CARTESIAN_POINT('Ctrl Pts',(-4.66090400079055,-9.19999999995039,
119.363676940337)) ;
#113768=CARTESIAN_POINT('Ctrl Pts',(-5.15142595671263,-9.04999999995038,
119.005623523177)) ;
#113769=CARTESIAN_POINT('Ctrl Pts',(-5.07231914777193,-9.19999999995039,
118.859385893862)) ;
#113770=CARTESIAN_POINT('Ctrl Pts',(-5.99494321694567,-9.04999999995039,
118.917647559852)) ;
#113771=CARTESIAN_POINT('Ctrl Pts',(-6.04236399869572,-9.19999999995039,
118.758213536859)) ;
#113772=CARTESIAN_POINT('Ctrl Pts',(-6.65417591390635,-9.04999999995041,
119.452805846097)) ;
#113773=CARTESIAN_POINT('Ctrl Pts',(-6.80048159967586,-9.19999999995041,
119.373645566077)) ;
#113774=CARTESIAN_POINT('Ctrl Pts',(-6.74142583978821,-9.0499999999504,
120.296857264431)) ;
#113775=CARTESIAN_POINT('Ctrl Pts',(-6.90081901473353,-9.1999999999504,
120.344304696983)) ;
#113776=CARTESIAN_POINT('Ctrl Pts',(-6.2067761094534,-9.04999999995039,
120.955784431796)) ;
#113777=CARTESIAN_POINT('Ctrl Pts',(-6.28597182491173,-9.19999999995039,
121.102070939682)) ;
#113778=CARTESIAN_POINT('Ctrl Pts',(-5.36219077623412,-9.04999999995039,
121.043293031702)) ;
#113779=CARTESIAN_POINT('Ctrl Pts',(-5.31469869100537,-9.19999999995039,
121.202705829313)) ;
#113780=CARTESIAN_POINT('Ctrl Pts',(-4.70410787109404,-9.04999999995041,
120.508327585707)) ;
#113781=CARTESIAN_POINT('Ctrl Pts',(-4.55790335108104,-9.1999999999504,
120.587495567235)) ;
#113782=CARTESIAN_POINT('Ctrl Pts',(-4.64441529656359,-9.0499999999504,
119.945550548028)) ;
#113783=CARTESIAN_POINT('Ctrl Pts',(-4.48925688934139,-9.19999999995039,
119.940301972492)) ;
#113784=CARTESIAN_POINT('Ctrl Pts',(-4.72036737313531,-9.0499999999504,
119.695237805925)) ;
#113785=CARTESIAN_POINT('Ctrl Pts',(-4.57660177482253,-9.1999999999504,
119.652442318957)) ;
#113786=CARTESIAN_POINT('',(-4.72036737313531,-9.0499999999504,119.695237805925)) ;
#196737=UNCERTAINTY_MEASURE_WITH_UNIT(LENGTH_MEASURE(0.01),#196742,
'DISTANCE_ACCURACY_VALUE',
'Maximum model space distance between geometric entities at asserted c
onnectivities') ;
#196738=UNCERTAINTY_MEASURE_WITH_UNIT(LENGTH_MEASURE(0.01),#196742,
'DISTANCE_ACCURACY_VALUE',
'Maximum model space distance between geometric entities at asserted c
onnectivities') ;
#196740=(
GEOMETRIC_REPRESENTATION_CONTEXT(3)
GLOBAL_UNCERTAINTY_ASSIGNED_CONTEXT((#196737))
GLOBAL_UNIT_ASSIGNED_CONTEXT((#196742,#196744,#196745))
REPRESENTATION_CONTEXT('','3D')
) ;
#196741=(
GEOMETRIC_REPRESENTATION_CONTEXT(3)
GLOBAL_UNCERTAINTY_ASSIGNED_CONTEXT((#196738))
GLOBAL_UNIT_ASSIGNED_CONTEXT((#196742,#196744,#196745))
REPRESENTATION_CONTEXT('','3D')
) ;
#196742=(
LENGTH_UNIT()
NAMED_UNIT(*)
SI_UNIT(.MILLI.,.METRE.)
) ;
#196744=(
NAMED_UNIT(*)
PLANE_ANGLE_UNIT()
SI_UNIT($,.RADIAN.)
) ;
#196745=(
NAMED_UNIT(*)
SI_UNIT($,.STERADIAN.)
SOLID_ANGLE_UNIT()
) ;
#196753=PRODUCT_DEFINITION_CONTEXT('part definition',#196761,'design') ;
#196761=APPLICATION_CONTEXT(
'Core Data for Automotive Mechanical Design Process') ;
#196762=PRODUCT_CONTEXT('part definition',#196761,'mechanical') ;
#196765=PRESENTATION_STYLE_ASSIGNMENT((#196767)) ;
#196767=SURFACE_STYLE_USAGE(.BOTH.,#196769) ;
#196769=SURFACE_SIDE_STYLE('',(#196771)) ;
#196771=SURFACE_STYLE_FILL_AREA(#196773) ;
#196773=FILL_AREA_STYLE('Steel - Satin',(#196775)) ;
#196775=FILL_AREA_STYLE_COLOUR('Steel - Satin',#196777) ;
#196777=COLOUR_RGB('Steel - Satin', 0.09019608, 0.27058824, 0.51372549) ;
#196947=CARTESIAN_POINT ( '', ( 0.0, 0.0, 0.0 ) ) ;
#196948=DIRECTION ( '', ( 0.0, 0.0, 1.0 ) ) ;
#196949=DIRECTION ( '', ( 1.0, 0.0, 0.0 ) ) ;
#196950=AXIS2_PLACEMENT_3D ( '', #196947, #196948, #196949 ) ;
#196951=ADVANCED_BREP_SHAPE_REPRESENTATION ( 'Exit Pallet Arm', ( #345, #196950, #196961, #197329 ), #196740 ) ;
#196952=PRODUCT( 'Exit Pallet Arm', 'Exit Pallet Arm', '', ( #196762 ) ) ;
#196953=PRODUCT_DEFINITION_FORMATION ( '', '', #196952 ) ;
#196954=PRODUCT_DEFINITION( 'Exit Pallet Arm', 'Exit Pallet Arm', #196953, #196753 ) ;
#196955=PRODUCT_DEFINITION_SHAPE ( '', '', #196954 ) ;
#196956=SHAPE_DEFINITION_REPRESENTATION ( #196955, #196951 ) ;
#196958=CARTESIAN_POINT ( '', ( 0.0, 0.0, 0.0 ) ) ;
#196959=DIRECTION ( '', ( 0.0, 0.0, 1.0 ) ) ;
#196960=DIRECTION ( '', ( 1.0, 0.0, 0.0 ) ) ;
#196961=AXIS2_PLACEMENT_3D ( '', #196958, #196959, #196960 ) ;
#197326=CARTESIAN_POINT ( '', ( 0.0, 0.0, 0.0 ) ) ;
#197327=DIRECTION ( '', ( 0.0, 0.0, 1.0 ) ) ;
#197328=DIRECTION ( '', ( 1.0, 0.0, 0.0 ) ) ;
#197329=AXIS2_PLACEMENT_3D ( '', #197326, #197327, #197328 ) ;
ENDSEC;
END-ISO-10303-21;
